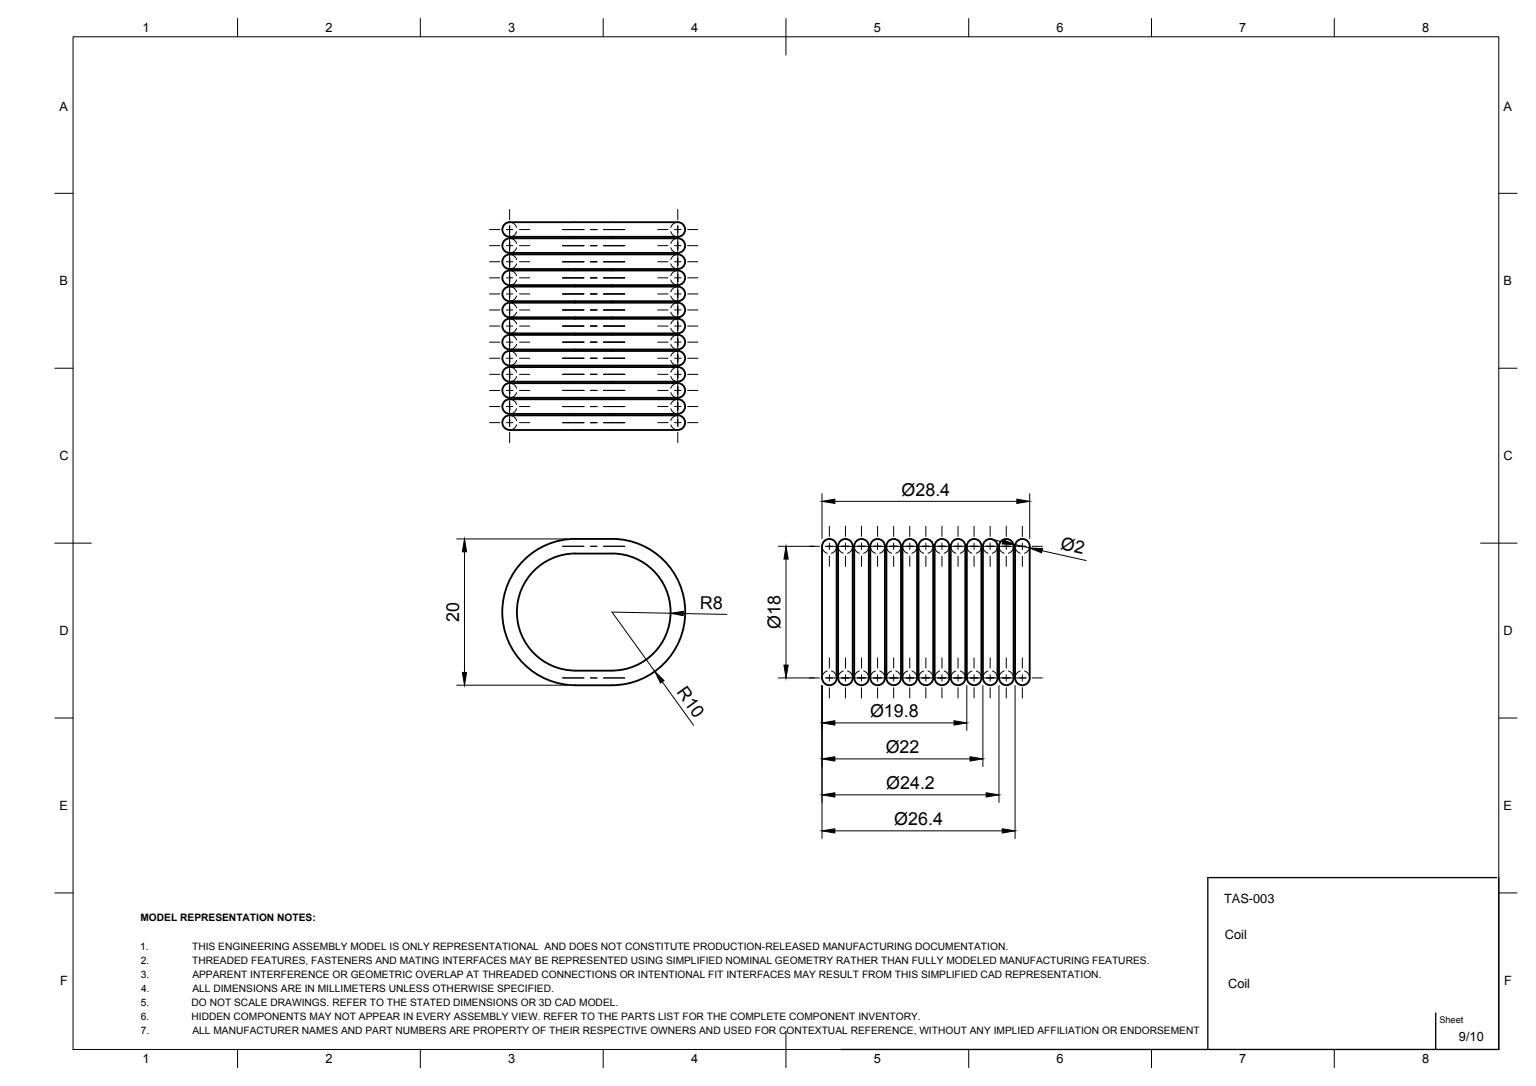
ISO-10303-21;
HEADER;
/* Generated by software containing ST-Developer
 * from STEP Tools, Inc. (www.steptools.com) 
 */

FILE_DESCRIPTION(
/* description */ ('STEP AP214'),
/* implementation_level */ '2;1');

FILE_NAME(
/* name */ 'coil.step',
/* time_stamp */ '2026-11-04T19:43:37-08:00',
/* author */ (''),
/* organization */ (''),
/* preprocessor_version */ 'ST-DEVELOPER v20.2',
/* originating_system */ 'Autodesk Translation Framework v15.17.0.0',
/* authorisation */ '');

FILE_SCHEMA (('AUTOMOTIVE_DESIGN { 1 0 10303 214 3 1 1 }'));
ENDSEC;

DATA;
#10=MECHANICAL_DESIGN_GEOMETRIC_PRESENTATION_REPRESENTATION('',(#121,#122,#123,#124,#125,#126,#127,#128,#129,#130,#131,#132,#133),#7627);
#60=TOROIDAL_SURFACE('',#2646,9.,0.999999999999999);
#61=TOROIDAL_SURFACE('',#2650,9.,0.999999999999999);
#62=TOROIDAL_SURFACE('',#2656,9.,0.999999999999999);
#63=TOROIDAL_SURFACE('',#2660,9.,0.999999999999999);
#64=TOROIDAL_SURFACE('',#2666,9.,0.999999999999999);
#65=TOROIDAL_SURFACE('',#2670,9.,0.999999999999999);
#66=TOROIDAL_SURFACE('',#2676,9.,0.999999999999999);
#67=TOROIDAL_SURFACE('',#2680,9.,0.999999999999999);
#68=TOROIDAL_SURFACE('',#2686,9.,0.999999999999999);
#69=TOROIDAL_SURFACE('',#2690,9.,0.999999999999999);
#70=TOROIDAL_SURFACE('',#2696,9.,0.999999999999999);
#71=TOROIDAL_SURFACE('',#2700,9.,0.999999999999999);
#72=TOROIDAL_SURFACE('',#2706,9.,0.999999999999999);
#73=TOROIDAL_SURFACE('',#2710,9.,0.999999999999999);
#74=TOROIDAL_SURFACE('',#2716,9.,0.999999999999999);
#75=TOROIDAL_SURFACE('',#2720,9.,0.999999999999999);
#76=TOROIDAL_SURFACE('',#2726,9.,0.999999999999999);
#77=TOROIDAL_SURFACE('',#2730,9.,0.999999999999999);
#78=TOROIDAL_SURFACE('',#2736,9.,0.999999999999999);
#79=TOROIDAL_SURFACE('',#2740,9.,0.999999999999999);
#80=TOROIDAL_SURFACE('',#2746,9.,0.999999999999999);
#81=TOROIDAL_SURFACE('',#2750,9.,0.999999999999999);
#82=TOROIDAL_SURFACE('',#2756,9.,0.999999999999999);
#83=TOROIDAL_SURFACE('',#2760,9.,0.999999999999999);
#84=TOROIDAL_SURFACE('',#2766,9.,0.999999999999999);
#85=TOROIDAL_SURFACE('',#2770,9.,0.999999999999999);
#103=SHAPE_REPRESENTATION_RELATIONSHIP('SRR','None',#7671,#112);
#112=ADVANCED_BREP_SHAPE_REPRESENTATION('',(#142,#143,#144,#145,#146,#147,
#148,#149,#150,#151,#152,#153,#154),#7624);
#121=STYLED_ITEM('',(#7723),#142);
#122=STYLED_ITEM('',(#7723),#143);
#123=STYLED_ITEM('',(#7723),#144);
#124=STYLED_ITEM('',(#7723),#145);
#125=STYLED_ITEM('',(#7723),#146);
#126=STYLED_ITEM('',(#7723),#147);
#127=STYLED_ITEM('',(#7723),#148);
#128=STYLED_ITEM('',(#7723),#149);
#129=STYLED_ITEM('',(#7723),#150);
#130=STYLED_ITEM('',(#7723),#151);
#131=STYLED_ITEM('',(#7723),#152);
#132=STYLED_ITEM('',(#7723),#153);
#133=STYLED_ITEM('',(#7723),#154);
#142=MANIFOLD_SOLID_BREP('Body1',#2419);
#143=MANIFOLD_SOLID_BREP('Body2',#2420);
#144=MANIFOLD_SOLID_BREP('Body3',#2421);
#145=MANIFOLD_SOLID_BREP('Body4',#2422);
#146=MANIFOLD_SOLID_BREP('Body5',#2423);
#147=MANIFOLD_SOLID_BREP('Body6',#2424);
#148=MANIFOLD_SOLID_BREP('Body7',#2425);
#149=MANIFOLD_SOLID_BREP('Body8',#2426);
#150=MANIFOLD_SOLID_BREP('Body9',#2427);
#151=MANIFOLD_SOLID_BREP('Body10',#2428);
#152=MANIFOLD_SOLID_BREP('Body11',#2429);
#153=MANIFOLD_SOLID_BREP('Body12',#2430);
#154=MANIFOLD_SOLID_BREP('Body13',#2431);
#276=CYLINDRICAL_SURFACE('',#2654,0.999999999999999);
#277=CYLINDRICAL_SURFACE('',#2655,0.999999999999999);
#278=CYLINDRICAL_SURFACE('',#2664,0.999999999999999);
#279=CYLINDRICAL_SURFACE('',#2665,0.999999999999999);
#280=CYLINDRICAL_SURFACE('',#2674,0.999999999999999);
#281=CYLINDRICAL_SURFACE('',#2675,0.999999999999999);
#282=CYLINDRICAL_SURFACE('',#2684,0.999999999999999);
#283=CYLINDRICAL_SURFACE('',#2685,0.999999999999999);
#284=CYLINDRICAL_SURFACE('',#2694,0.999999999999999);
#285=CYLINDRICAL_SURFACE('',#2695,0.999999999999999);
#286=CYLINDRICAL_SURFACE('',#2704,0.999999999999999);
#287=CYLINDRICAL_SURFACE('',#2705,0.999999999999999);
#288=CYLINDRICAL_SURFACE('',#2714,0.999999999999999);
#289=CYLINDRICAL_SURFACE('',#2715,0.999999999999999);
#290=CYLINDRICAL_SURFACE('',#2724,0.999999999999999);
#291=CYLINDRICAL_SURFACE('',#2725,0.999999999999999);
#292=CYLINDRICAL_SURFACE('',#2734,0.999999999999999);
#293=CYLINDRICAL_SURFACE('',#2735,0.999999999999999);
#294=CYLINDRICAL_SURFACE('',#2744,0.999999999999999);
#295=CYLINDRICAL_SURFACE('',#2745,0.999999999999999);
#296=CYLINDRICAL_SURFACE('',#2754,0.999999999999999);
#297=CYLINDRICAL_SURFACE('',#2755,0.999999999999999);
#298=CYLINDRICAL_SURFACE('',#2764,0.999999999999999);
#299=CYLINDRICAL_SURFACE('',#2765,0.999999999999999);
#300=CYLINDRICAL_SURFACE('',#2774,0.999999999999999);
#301=CYLINDRICAL_SURFACE('',#2775,0.999999999999999);
#366=FACE_OUTER_BOUND('',#542,.T.);
#367=FACE_OUTER_BOUND('',#543,.T.);
#368=FACE_OUTER_BOUND('',#544,.T.);
#369=FACE_OUTER_BOUND('',#545,.T.);
#370=FACE_OUTER_BOUND('',#546,.T.);
#371=FACE_OUTER_BOUND('',#547,.T.);
#372=FACE_OUTER_BOUND('',#548,.T.);
#373=FACE_OUTER_BOUND('',#549,.T.);
#374=FACE_OUTER_BOUND('',#550,.T.);
#375=FACE_OUTER_BOUND('',#551,.T.);
#376=FACE_OUTER_BOUND('',#552,.T.);
#377=FACE_OUTER_BOUND('',#553,.T.);
#378=FACE_OUTER_BOUND('',#554,.T.);
#379=FACE_OUTER_BOUND('',#555,.T.);
#380=FACE_OUTER_BOUND('',#556,.T.);
#381=FACE_OUTER_BOUND('',#557,.T.);
#382=FACE_OUTER_BOUND('',#558,.T.);
#383=FACE_OUTER_BOUND('',#559,.T.);
#384=FACE_OUTER_BOUND('',#560,.T.);
#385=FACE_OUTER_BOUND('',#561,.T.);
#386=FACE_OUTER_BOUND('',#562,.T.);
#387=FACE_OUTER_BOUND('',#563,.T.);
#388=FACE_OUTER_BOUND('',#564,.T.);
#389=FACE_OUTER_BOUND('',#565,.T.);
#390=FACE_OUTER_BOUND('',#566,.T.);
#391=FACE_OUTER_BOUND('',#567,.T.);
#392=FACE_OUTER_BOUND('',#568,.T.);
#393=FACE_OUTER_BOUND('',#569,.T.);
#394=FACE_OUTER_BOUND('',#570,.T.);
#395=FACE_OUTER_BOUND('',#571,.T.);
#396=FACE_OUTER_BOUND('',#572,.T.);
#397=FACE_OUTER_BOUND('',#573,.T.);
#398=FACE_OUTER_BOUND('',#574,.T.);
#399=FACE_OUTER_BOUND('',#575,.T.);
#400=FACE_OUTER_BOUND('',#576,.T.);
#401=FACE_OUTER_BOUND('',#577,.T.);
#402=FACE_OUTER_BOUND('',#578,.T.);
#403=FACE_OUTER_BOUND('',#579,.T.);
#404=FACE_OUTER_BOUND('',#580,.T.);
#405=FACE_OUTER_BOUND('',#581,.T.);
#406=FACE_OUTER_BOUND('',#582,.T.);
#407=FACE_OUTER_BOUND('',#583,.T.);
#408=FACE_OUTER_BOUND('',#584,.T.);
#409=FACE_OUTER_BOUND('',#585,.T.);
#410=FACE_OUTER_BOUND('',#586,.T.);
#411=FACE_OUTER_BOUND('',#587,.T.);
#412=FACE_OUTER_BOUND('',#588,.T.);
#413=FACE_OUTER_BOUND('',#589,.T.);
#414=FACE_OUTER_BOUND('',#590,.T.);
#415=FACE_OUTER_BOUND('',#591,.T.);
#416=FACE_OUTER_BOUND('',#592,.T.);
#417=FACE_OUTER_BOUND('',#593,.T.);
#542=EDGE_LOOP('',(#1849,#1850,#1851,#1852));
#543=EDGE_LOOP('',(#1853,#1854,#1855,#1856));
#544=EDGE_LOOP('',(#1857,#1858,#1859,#1860));
#545=EDGE_LOOP('',(#1861,#1862,#1863,#1864));
#546=EDGE_LOOP('',(#1865,#1866,#1867,#1868));
#547=EDGE_LOOP('',(#1869,#1870,#1871,#1872));
#548=EDGE_LOOP('',(#1873,#1874,#1875,#1876));
#549=EDGE_LOOP('',(#1877,#1878,#1879,#1880));
#550=EDGE_LOOP('',(#1881,#1882,#1883,#1884));
#551=EDGE_LOOP('',(#1885,#1886,#1887,#1888));
#552=EDGE_LOOP('',(#1889,#1890,#1891,#1892));
#553=EDGE_LOOP('',(#1893,#1894,#1895,#1896));
#554=EDGE_LOOP('',(#1897,#1898,#1899,#1900));
#555=EDGE_LOOP('',(#1901,#1902,#1903,#1904));
#556=EDGE_LOOP('',(#1905,#1906,#1907,#1908));
#557=EDGE_LOOP('',(#1909,#1910,#1911,#1912));
#558=EDGE_LOOP('',(#1913,#1914,#1915,#1916));
#559=EDGE_LOOP('',(#1917,#1918,#1919,#1920));
#560=EDGE_LOOP('',(#1921,#1922,#1923,#1924));
#561=EDGE_LOOP('',(#1925,#1926,#1927,#1928));
#562=EDGE_LOOP('',(#1929,#1930,#1931,#1932));
#563=EDGE_LOOP('',(#1933,#1934,#1935,#1936));
#564=EDGE_LOOP('',(#1937,#1938,#1939,#1940));
#565=EDGE_LOOP('',(#1941,#1942,#1943,#1944));
#566=EDGE_LOOP('',(#1945,#1946,#1947,#1948));
#567=EDGE_LOOP('',(#1949,#1950,#1951,#1952));
#568=EDGE_LOOP('',(#1953,#1954,#1955,#1956));
#569=EDGE_LOOP('',(#1957,#1958,#1959,#1960));
#570=EDGE_LOOP('',(#1961,#1962,#1963,#1964));
#571=EDGE_LOOP('',(#1965,#1966,#1967,#1968));
#572=EDGE_LOOP('',(#1969,#1970,#1971,#1972));
#573=EDGE_LOOP('',(#1973,#1974,#1975,#1976));
#574=EDGE_LOOP('',(#1977,#1978,#1979,#1980));
#575=EDGE_LOOP('',(#1981,#1982,#1983,#1984));
#576=EDGE_LOOP('',(#1985,#1986,#1987,#1988));
#577=EDGE_LOOP('',(#1989,#1990,#1991,#1992));
#578=EDGE_LOOP('',(#1993,#1994,#1995,#1996));
#579=EDGE_LOOP('',(#1997,#1998,#1999,#2000));
#580=EDGE_LOOP('',(#2001,#2002,#2003,#2004));
#581=EDGE_LOOP('',(#2005,#2006,#2007,#2008));
#582=EDGE_LOOP('',(#2009,#2010,#2011,#2012));
#583=EDGE_LOOP('',(#2013,#2014,#2015,#2016));
#584=EDGE_LOOP('',(#2017,#2018,#2019,#2020));
#585=EDGE_LOOP('',(#2021,#2022,#2023,#2024));
#586=EDGE_LOOP('',(#2025,#2026,#2027,#2028));
#587=EDGE_LOOP('',(#2029,#2030,#2031,#2032));
#588=EDGE_LOOP('',(#2033,#2034,#2035,#2036));
#589=EDGE_LOOP('',(#2037,#2038,#2039,#2040));
#590=EDGE_LOOP('',(#2041,#2042,#2043,#2044));
#591=EDGE_LOOP('',(#2045,#2046,#2047,#2048));
#592=EDGE_LOOP('',(#2049,#2050,#2051,#2052));
#593=EDGE_LOOP('',(#2053,#2054,#2055,#2056));
#695=CIRCLE('',#2647,0.999999999999999);
#696=CIRCLE('',#2648,8.00000000000001);
#697=CIRCLE('',#2649,0.999999999999999);
#698=CIRCLE('',#2651,0.999999999999999);
#699=CIRCLE('',#2652,8.);
#700=CIRCLE('',#2653,0.999999999999999);
#701=CIRCLE('',#2657,0.999999999999999);
#702=CIRCLE('',#2658,8.00000000000001);
#703=CIRCLE('',#2659,0.999999999999999);
#704=CIRCLE('',#2661,0.999999999999999);
#705=CIRCLE('',#2662,8.);
#706=CIRCLE('',#2663,0.999999999999999);
#707=CIRCLE('',#2667,0.999999999999999);
#708=CIRCLE('',#2668,8.00000000000001);
#709=CIRCLE('',#2669,0.999999999999999);
#710=CIRCLE('',#2671,0.999999999999999);
#711=CIRCLE('',#2672,8.);
#712=CIRCLE('',#2673,0.999999999999999);
#713=CIRCLE('',#2677,0.999999999999999);
#714=CIRCLE('',#2678,8.00000000000001);
#715=CIRCLE('',#2679,0.999999999999999);
#716=CIRCLE('',#2681,0.999999999999999);
#717=CIRCLE('',#2682,8.);
#718=CIRCLE('',#2683,0.999999999999999);
#719=CIRCLE('',#2687,0.999999999999999);
#720=CIRCLE('',#2688,8.00000000000001);
#721=CIRCLE('',#2689,0.999999999999999);
#722=CIRCLE('',#2691,0.999999999999999);
#723=CIRCLE('',#2692,8.);
#724=CIRCLE('',#2693,0.999999999999999);
#725=CIRCLE('',#2697,0.999999999999999);
#726=CIRCLE('',#2698,8.00000000000001);
#727=CIRCLE('',#2699,0.999999999999999);
#728=CIRCLE('',#2701,0.999999999999999);
#729=CIRCLE('',#2702,8.);
#730=CIRCLE('',#2703,0.999999999999999);
#731=CIRCLE('',#2707,0.999999999999999);
#732=CIRCLE('',#2708,8.00000000000001);
#733=CIRCLE('',#2709,0.999999999999999);
#734=CIRCLE('',#2711,0.999999999999999);
#735=CIRCLE('',#2712,8.);
#736=CIRCLE('',#2713,0.999999999999999);
#737=CIRCLE('',#2717,0.999999999999999);
#738=CIRCLE('',#2718,8.00000000000001);
#739=CIRCLE('',#2719,0.999999999999999);
#740=CIRCLE('',#2721,0.999999999999999);
#741=CIRCLE('',#2722,8.);
#742=CIRCLE('',#2723,0.999999999999999);
#743=CIRCLE('',#2727,0.999999999999999);
#744=CIRCLE('',#2728,8.00000000000001);
#745=CIRCLE('',#2729,0.999999999999999);
#746=CIRCLE('',#2731,0.999999999999999);
#747=CIRCLE('',#2732,8.);
#748=CIRCLE('',#2733,0.999999999999999);
#749=CIRCLE('',#2737,0.999999999999999);
#750=CIRCLE('',#2738,8.00000000000001);
#751=CIRCLE('',#2739,0.999999999999999);
#752=CIRCLE('',#2741,0.999999999999999);
#753=CIRCLE('',#2742,8.);
#754=CIRCLE('',#2743,0.999999999999999);
#755=CIRCLE('',#2747,0.999999999999999);
#756=CIRCLE('',#2748,8.00000000000001);
#757=CIRCLE('',#2749,0.999999999999999);
#758=CIRCLE('',#2751,0.999999999999999);
#759=CIRCLE('',#2752,8.);
#760=CIRCLE('',#2753,0.999999999999999);
#761=CIRCLE('',#2757,0.999999999999999);
#762=CIRCLE('',#2758,8.00000000000001);
#763=CIRCLE('',#2759,0.999999999999999);
#764=CIRCLE('',#2761,0.999999999999999);
#765=CIRCLE('',#2762,8.);
#766=CIRCLE('',#2763,0.999999999999999);
#767=CIRCLE('',#2767,0.999999999999999);
#768=CIRCLE('',#2768,8.00000000000001);
#769=CIRCLE('',#2769,0.999999999999999);
#770=CIRCLE('',#2771,0.999999999999999);
#771=CIRCLE('',#2772,8.);
#772=CIRCLE('',#2773,0.999999999999999);
#865=LINE('',#7193,#1021);
#866=LINE('',#7195,#1022);
#867=LINE('',#7209,#1023);
#868=LINE('',#7211,#1024);
#869=LINE('',#7225,#1025);
#870=LINE('',#7227,#1026);
#871=LINE('',#7241,#1027);
#872=LINE('',#7243,#1028);
#873=LINE('',#7257,#1029);
#874=LINE('',#7259,#1030);
#875=LINE('',#7273,#1031);
#876=LINE('',#7275,#1032);
#877=LINE('',#7289,#1033);
#878=LINE('',#7291,#1034);
#879=LINE('',#7305,#1035);
#880=LINE('',#7307,#1036);
#881=LINE('',#7321,#1037);
#882=LINE('',#7323,#1038);
#883=LINE('',#7337,#1039);
#884=LINE('',#7339,#1040);
#885=LINE('',#7353,#1041);
#886=LINE('',#7355,#1042);
#887=LINE('',#7369,#1043);
#888=LINE('',#7371,#1044);
#889=LINE('',#7385,#1045);
#890=LINE('',#7387,#1046);
#1021=VECTOR('',#3168,0.999999999999999);
#1022=VECTOR('',#3171,0.999999999999999);
#1023=VECTOR('',#3190,0.999999999999999);
#1024=VECTOR('',#3193,0.999999999999999);
#1025=VECTOR('',#3212,0.999999999999999);
#1026=VECTOR('',#3215,0.999999999999999);
#1027=VECTOR('',#3234,0.999999999999999);
#1028=VECTOR('',#3237,0.999999999999999);
#1029=VECTOR('',#3256,0.999999999999999);
#1030=VECTOR('',#3259,0.999999999999999);
#1031=VECTOR('',#3278,0.999999999999999);
#1032=VECTOR('',#3281,0.999999999999999);
#1033=VECTOR('',#3300,0.999999999999999);
#1034=VECTOR('',#3303,0.999999999999999);
#1035=VECTOR('',#3322,0.999999999999999);
#1036=VECTOR('',#3325,0.999999999999999);
#1037=VECTOR('',#3344,0.999999999999999);
#1038=VECTOR('',#3347,0.999999999999999);
#1039=VECTOR('',#3366,0.999999999999999);
#1040=VECTOR('',#3369,0.999999999999999);
#1041=VECTOR('',#3388,0.999999999999999);
#1042=VECTOR('',#3391,0.999999999999999);
#1043=VECTOR('',#3410,0.999999999999999);
#1044=VECTOR('',#3413,0.999999999999999);
#1045=VECTOR('',#3432,0.999999999999999);
#1046=VECTOR('',#3435,0.999999999999999);
#1191=VERTEX_POINT('',#7181);
#1192=VERTEX_POINT('',#7183);
#1193=VERTEX_POINT('',#7187);
#1194=VERTEX_POINT('',#7189);
#1195=VERTEX_POINT('',#7197);
#1196=VERTEX_POINT('',#7199);
#1197=VERTEX_POINT('',#7203);
#1198=VERTEX_POINT('',#7205);
#1199=VERTEX_POINT('',#7213);
#1200=VERTEX_POINT('',#7215);
#1201=VERTEX_POINT('',#7219);
#1202=VERTEX_POINT('',#7221);
#1203=VERTEX_POINT('',#7229);
#1204=VERTEX_POINT('',#7231);
#1205=VERTEX_POINT('',#7235);
#1206=VERTEX_POINT('',#7237);
#1207=VERTEX_POINT('',#7245);
#1208=VERTEX_POINT('',#7247);
#1209=VERTEX_POINT('',#7251);
#1210=VERTEX_POINT('',#7253);
#1211=VERTEX_POINT('',#7261);
#1212=VERTEX_POINT('',#7263);
#1213=VERTEX_POINT('',#7267);
#1214=VERTEX_POINT('',#7269);
#1215=VERTEX_POINT('',#7277);
#1216=VERTEX_POINT('',#7279);
#1217=VERTEX_POINT('',#7283);
#1218=VERTEX_POINT('',#7285);
#1219=VERTEX_POINT('',#7293);
#1220=VERTEX_POINT('',#7295);
#1221=VERTEX_POINT('',#7299);
#1222=VERTEX_POINT('',#7301);
#1223=VERTEX_POINT('',#7309);
#1224=VERTEX_POINT('',#7311);
#1225=VERTEX_POINT('',#7315);
#1226=VERTEX_POINT('',#7317);
#1227=VERTEX_POINT('',#7325);
#1228=VERTEX_POINT('',#7327);
#1229=VERTEX_POINT('',#7331);
#1230=VERTEX_POINT('',#7333);
#1231=VERTEX_POINT('',#7341);
#1232=VERTEX_POINT('',#7343);
#1233=VERTEX_POINT('',#7347);
#1234=VERTEX_POINT('',#7349);
#1235=VERTEX_POINT('',#7357);
#1236=VERTEX_POINT('',#7359);
#1237=VERTEX_POINT('',#7363);
#1238=VERTEX_POINT('',#7365);
#1239=VERTEX_POINT('',#7373);
#1240=VERTEX_POINT('',#7375);
#1241=VERTEX_POINT('',#7379);
#1242=VERTEX_POINT('',#7381);
#1419=EDGE_CURVE('',#1191,#1191,#695,.T.);
#1420=EDGE_CURVE('',#1191,#1192,#696,.T.);
#1421=EDGE_CURVE('',#1192,#1192,#697,.T.);
#1422=EDGE_CURVE('',#1193,#1193,#698,.T.);
#1423=EDGE_CURVE('',#1193,#1194,#699,.T.);
#1424=EDGE_CURVE('',#1194,#1194,#700,.T.);
#1425=EDGE_CURVE('',#1194,#1191,#865,.T.);
#1426=EDGE_CURVE('',#1192,#1193,#866,.T.);
#1427=EDGE_CURVE('',#1195,#1195,#701,.T.);
#1428=EDGE_CURVE('',#1195,#1196,#702,.T.);
#1429=EDGE_CURVE('',#1196,#1196,#703,.T.);
#1430=EDGE_CURVE('',#1197,#1197,#704,.T.);
#1431=EDGE_CURVE('',#1197,#1198,#705,.T.);
#1432=EDGE_CURVE('',#1198,#1198,#706,.T.);
#1433=EDGE_CURVE('',#1198,#1195,#867,.T.);
#1434=EDGE_CURVE('',#1196,#1197,#868,.T.);
#1435=EDGE_CURVE('',#1199,#1199,#707,.T.);
#1436=EDGE_CURVE('',#1199,#1200,#708,.T.);
#1437=EDGE_CURVE('',#1200,#1200,#709,.T.);
#1438=EDGE_CURVE('',#1201,#1201,#710,.T.);
#1439=EDGE_CURVE('',#1201,#1202,#711,.T.);
#1440=EDGE_CURVE('',#1202,#1202,#712,.T.);
#1441=EDGE_CURVE('',#1202,#1199,#869,.T.);
#1442=EDGE_CURVE('',#1200,#1201,#870,.T.);
#1443=EDGE_CURVE('',#1203,#1203,#713,.T.);
#1444=EDGE_CURVE('',#1203,#1204,#714,.T.);
#1445=EDGE_CURVE('',#1204,#1204,#715,.T.);
#1446=EDGE_CURVE('',#1205,#1205,#716,.T.);
#1447=EDGE_CURVE('',#1205,#1206,#717,.T.);
#1448=EDGE_CURVE('',#1206,#1206,#718,.T.);
#1449=EDGE_CURVE('',#1206,#1203,#871,.T.);
#1450=EDGE_CURVE('',#1204,#1205,#872,.T.);
#1451=EDGE_CURVE('',#1207,#1207,#719,.T.);
#1452=EDGE_CURVE('',#1207,#1208,#720,.T.);
#1453=EDGE_CURVE('',#1208,#1208,#721,.T.);
#1454=EDGE_CURVE('',#1209,#1209,#722,.T.);
#1455=EDGE_CURVE('',#1209,#1210,#723,.T.);
#1456=EDGE_CURVE('',#1210,#1210,#724,.T.);
#1457=EDGE_CURVE('',#1210,#1207,#873,.T.);
#1458=EDGE_CURVE('',#1208,#1209,#874,.T.);
#1459=EDGE_CURVE('',#1211,#1211,#725,.T.);
#1460=EDGE_CURVE('',#1211,#1212,#726,.T.);
#1461=EDGE_CURVE('',#1212,#1212,#727,.T.);
#1462=EDGE_CURVE('',#1213,#1213,#728,.T.);
#1463=EDGE_CURVE('',#1213,#1214,#729,.T.);
#1464=EDGE_CURVE('',#1214,#1214,#730,.T.);
#1465=EDGE_CURVE('',#1214,#1211,#875,.T.);
#1466=EDGE_CURVE('',#1212,#1213,#876,.T.);
#1467=EDGE_CURVE('',#1215,#1215,#731,.T.);
#1468=EDGE_CURVE('',#1215,#1216,#732,.T.);
#1469=EDGE_CURVE('',#1216,#1216,#733,.T.);
#1470=EDGE_CURVE('',#1217,#1217,#734,.T.);
#1471=EDGE_CURVE('',#1217,#1218,#735,.T.);
#1472=EDGE_CURVE('',#1218,#1218,#736,.T.);
#1473=EDGE_CURVE('',#1218,#1215,#877,.T.);
#1474=EDGE_CURVE('',#1216,#1217,#878,.T.);
#1475=EDGE_CURVE('',#1219,#1219,#737,.T.);
#1476=EDGE_CURVE('',#1219,#1220,#738,.T.);
#1477=EDGE_CURVE('',#1220,#1220,#739,.T.);
#1478=EDGE_CURVE('',#1221,#1221,#740,.T.);
#1479=EDGE_CURVE('',#1221,#1222,#741,.T.);
#1480=EDGE_CURVE('',#1222,#1222,#742,.T.);
#1481=EDGE_CURVE('',#1222,#1219,#879,.T.);
#1482=EDGE_CURVE('',#1220,#1221,#880,.T.);
#1483=EDGE_CURVE('',#1223,#1223,#743,.T.);
#1484=EDGE_CURVE('',#1223,#1224,#744,.T.);
#1485=EDGE_CURVE('',#1224,#1224,#745,.T.);
#1486=EDGE_CURVE('',#1225,#1225,#746,.T.);
#1487=EDGE_CURVE('',#1225,#1226,#747,.T.);
#1488=EDGE_CURVE('',#1226,#1226,#748,.T.);
#1489=EDGE_CURVE('',#1226,#1223,#881,.T.);
#1490=EDGE_CURVE('',#1224,#1225,#882,.T.);
#1491=EDGE_CURVE('',#1227,#1227,#749,.T.);
#1492=EDGE_CURVE('',#1227,#1228,#750,.T.);
#1493=EDGE_CURVE('',#1228,#1228,#751,.T.);
#1494=EDGE_CURVE('',#1229,#1229,#752,.T.);
#1495=EDGE_CURVE('',#1229,#1230,#753,.T.);
#1496=EDGE_CURVE('',#1230,#1230,#754,.T.);
#1497=EDGE_CURVE('',#1230,#1227,#883,.T.);
#1498=EDGE_CURVE('',#1228,#1229,#884,.T.);
#1499=EDGE_CURVE('',#1231,#1231,#755,.T.);
#1500=EDGE_CURVE('',#1231,#1232,#756,.T.);
#1501=EDGE_CURVE('',#1232,#1232,#757,.T.);
#1502=EDGE_CURVE('',#1233,#1233,#758,.T.);
#1503=EDGE_CURVE('',#1233,#1234,#759,.T.);
#1504=EDGE_CURVE('',#1234,#1234,#760,.T.);
#1505=EDGE_CURVE('',#1234,#1231,#885,.T.);
#1506=EDGE_CURVE('',#1232,#1233,#886,.T.);
#1507=EDGE_CURVE('',#1235,#1235,#761,.T.);
#1508=EDGE_CURVE('',#1235,#1236,#762,.T.);
#1509=EDGE_CURVE('',#1236,#1236,#763,.T.);
#1510=EDGE_CURVE('',#1237,#1237,#764,.T.);
#1511=EDGE_CURVE('',#1237,#1238,#765,.T.);
#1512=EDGE_CURVE('',#1238,#1238,#766,.T.);
#1513=EDGE_CURVE('',#1238,#1235,#887,.T.);
#1514=EDGE_CURVE('',#1236,#1237,#888,.T.);
#1515=EDGE_CURVE('',#1239,#1239,#767,.T.);
#1516=EDGE_CURVE('',#1239,#1240,#768,.T.);
#1517=EDGE_CURVE('',#1240,#1240,#769,.T.);
#1518=EDGE_CURVE('',#1241,#1241,#770,.T.);
#1519=EDGE_CURVE('',#1241,#1242,#771,.T.);
#1520=EDGE_CURVE('',#1242,#1242,#772,.T.);
#1521=EDGE_CURVE('',#1242,#1239,#889,.T.);
#1522=EDGE_CURVE('',#1240,#1241,#890,.T.);
#1849=ORIENTED_EDGE('',*,*,#1419,.T.);
#1850=ORIENTED_EDGE('',*,*,#1420,.T.);
#1851=ORIENTED_EDGE('',*,*,#1421,.F.);
#1852=ORIENTED_EDGE('',*,*,#1420,.F.);
#1853=ORIENTED_EDGE('',*,*,#1422,.T.);
#1854=ORIENTED_EDGE('',*,*,#1423,.T.);
#1855=ORIENTED_EDGE('',*,*,#1424,.F.);
#1856=ORIENTED_EDGE('',*,*,#1423,.F.);
#1857=ORIENTED_EDGE('',*,*,#1424,.T.);
#1858=ORIENTED_EDGE('',*,*,#1425,.T.);
#1859=ORIENTED_EDGE('',*,*,#1419,.F.);
#1860=ORIENTED_EDGE('',*,*,#1425,.F.);
#1861=ORIENTED_EDGE('',*,*,#1421,.T.);
#1862=ORIENTED_EDGE('',*,*,#1426,.T.);
#1863=ORIENTED_EDGE('',*,*,#1422,.F.);
#1864=ORIENTED_EDGE('',*,*,#1426,.F.);
#1865=ORIENTED_EDGE('',*,*,#1427,.T.);
#1866=ORIENTED_EDGE('',*,*,#1428,.T.);
#1867=ORIENTED_EDGE('',*,*,#1429,.F.);
#1868=ORIENTED_EDGE('',*,*,#1428,.F.);
#1869=ORIENTED_EDGE('',*,*,#1430,.T.);
#1870=ORIENTED_EDGE('',*,*,#1431,.T.);
#1871=ORIENTED_EDGE('',*,*,#1432,.F.);
#1872=ORIENTED_EDGE('',*,*,#1431,.F.);
#1873=ORIENTED_EDGE('',*,*,#1432,.T.);
#1874=ORIENTED_EDGE('',*,*,#1433,.T.);
#1875=ORIENTED_EDGE('',*,*,#1427,.F.);
#1876=ORIENTED_EDGE('',*,*,#1433,.F.);
#1877=ORIENTED_EDGE('',*,*,#1429,.T.);
#1878=ORIENTED_EDGE('',*,*,#1434,.T.);
#1879=ORIENTED_EDGE('',*,*,#1430,.F.);
#1880=ORIENTED_EDGE('',*,*,#1434,.F.);
#1881=ORIENTED_EDGE('',*,*,#1435,.T.);
#1882=ORIENTED_EDGE('',*,*,#1436,.T.);
#1883=ORIENTED_EDGE('',*,*,#1437,.F.);
#1884=ORIENTED_EDGE('',*,*,#1436,.F.);
#1885=ORIENTED_EDGE('',*,*,#1438,.T.);
#1886=ORIENTED_EDGE('',*,*,#1439,.T.);
#1887=ORIENTED_EDGE('',*,*,#1440,.F.);
#1888=ORIENTED_EDGE('',*,*,#1439,.F.);
#1889=ORIENTED_EDGE('',*,*,#1440,.T.);
#1890=ORIENTED_EDGE('',*,*,#1441,.T.);
#1891=ORIENTED_EDGE('',*,*,#1435,.F.);
#1892=ORIENTED_EDGE('',*,*,#1441,.F.);
#1893=ORIENTED_EDGE('',*,*,#1437,.T.);
#1894=ORIENTED_EDGE('',*,*,#1442,.T.);
#1895=ORIENTED_EDGE('',*,*,#1438,.F.);
#1896=ORIENTED_EDGE('',*,*,#1442,.F.);
#1897=ORIENTED_EDGE('',*,*,#1443,.T.);
#1898=ORIENTED_EDGE('',*,*,#1444,.T.);
#1899=ORIENTED_EDGE('',*,*,#1445,.F.);
#1900=ORIENTED_EDGE('',*,*,#1444,.F.);
#1901=ORIENTED_EDGE('',*,*,#1446,.T.);
#1902=ORIENTED_EDGE('',*,*,#1447,.T.);
#1903=ORIENTED_EDGE('',*,*,#1448,.F.);
#1904=ORIENTED_EDGE('',*,*,#1447,.F.);
#1905=ORIENTED_EDGE('',*,*,#1448,.T.);
#1906=ORIENTED_EDGE('',*,*,#1449,.T.);
#1907=ORIENTED_EDGE('',*,*,#1443,.F.);
#1908=ORIENTED_EDGE('',*,*,#1449,.F.);
#1909=ORIENTED_EDGE('',*,*,#1445,.T.);
#1910=ORIENTED_EDGE('',*,*,#1450,.T.);
#1911=ORIENTED_EDGE('',*,*,#1446,.F.);
#1912=ORIENTED_EDGE('',*,*,#1450,.F.);
#1913=ORIENTED_EDGE('',*,*,#1451,.T.);
#1914=ORIENTED_EDGE('',*,*,#1452,.T.);
#1915=ORIENTED_EDGE('',*,*,#1453,.F.);
#1916=ORIENTED_EDGE('',*,*,#1452,.F.);
#1917=ORIENTED_EDGE('',*,*,#1454,.T.);
#1918=ORIENTED_EDGE('',*,*,#1455,.T.);
#1919=ORIENTED_EDGE('',*,*,#1456,.F.);
#1920=ORIENTED_EDGE('',*,*,#1455,.F.);
#1921=ORIENTED_EDGE('',*,*,#1456,.T.);
#1922=ORIENTED_EDGE('',*,*,#1457,.T.);
#1923=ORIENTED_EDGE('',*,*,#1451,.F.);
#1924=ORIENTED_EDGE('',*,*,#1457,.F.);
#1925=ORIENTED_EDGE('',*,*,#1453,.T.);
#1926=ORIENTED_EDGE('',*,*,#1458,.T.);
#1927=ORIENTED_EDGE('',*,*,#1454,.F.);
#1928=ORIENTED_EDGE('',*,*,#1458,.F.);
#1929=ORIENTED_EDGE('',*,*,#1459,.T.);
#1930=ORIENTED_EDGE('',*,*,#1460,.T.);
#1931=ORIENTED_EDGE('',*,*,#1461,.F.);
#1932=ORIENTED_EDGE('',*,*,#1460,.F.);
#1933=ORIENTED_EDGE('',*,*,#1462,.T.);
#1934=ORIENTED_EDGE('',*,*,#1463,.T.);
#1935=ORIENTED_EDGE('',*,*,#1464,.F.);
#1936=ORIENTED_EDGE('',*,*,#1463,.F.);
#1937=ORIENTED_EDGE('',*,*,#1464,.T.);
#1938=ORIENTED_EDGE('',*,*,#1465,.T.);
#1939=ORIENTED_EDGE('',*,*,#1459,.F.);
#1940=ORIENTED_EDGE('',*,*,#1465,.F.);
#1941=ORIENTED_EDGE('',*,*,#1461,.T.);
#1942=ORIENTED_EDGE('',*,*,#1466,.T.);
#1943=ORIENTED_EDGE('',*,*,#1462,.F.);
#1944=ORIENTED_EDGE('',*,*,#1466,.F.);
#1945=ORIENTED_EDGE('',*,*,#1467,.T.);
#1946=ORIENTED_EDGE('',*,*,#1468,.T.);
#1947=ORIENTED_EDGE('',*,*,#1469,.F.);
#1948=ORIENTED_EDGE('',*,*,#1468,.F.);
#1949=ORIENTED_EDGE('',*,*,#1470,.T.);
#1950=ORIENTED_EDGE('',*,*,#1471,.T.);
#1951=ORIENTED_EDGE('',*,*,#1472,.F.);
#1952=ORIENTED_EDGE('',*,*,#1471,.F.);
#1953=ORIENTED_EDGE('',*,*,#1472,.T.);
#1954=ORIENTED_EDGE('',*,*,#1473,.T.);
#1955=ORIENTED_EDGE('',*,*,#1467,.F.);
#1956=ORIENTED_EDGE('',*,*,#1473,.F.);
#1957=ORIENTED_EDGE('',*,*,#1469,.T.);
#1958=ORIENTED_EDGE('',*,*,#1474,.T.);
#1959=ORIENTED_EDGE('',*,*,#1470,.F.);
#1960=ORIENTED_EDGE('',*,*,#1474,.F.);
#1961=ORIENTED_EDGE('',*,*,#1475,.T.);
#1962=ORIENTED_EDGE('',*,*,#1476,.T.);
#1963=ORIENTED_EDGE('',*,*,#1477,.F.);
#1964=ORIENTED_EDGE('',*,*,#1476,.F.);
#1965=ORIENTED_EDGE('',*,*,#1478,.T.);
#1966=ORIENTED_EDGE('',*,*,#1479,.T.);
#1967=ORIENTED_EDGE('',*,*,#1480,.F.);
#1968=ORIENTED_EDGE('',*,*,#1479,.F.);
#1969=ORIENTED_EDGE('',*,*,#1480,.T.);
#1970=ORIENTED_EDGE('',*,*,#1481,.T.);
#1971=ORIENTED_EDGE('',*,*,#1475,.F.);
#1972=ORIENTED_EDGE('',*,*,#1481,.F.);
#1973=ORIENTED_EDGE('',*,*,#1477,.T.);
#1974=ORIENTED_EDGE('',*,*,#1482,.T.);
#1975=ORIENTED_EDGE('',*,*,#1478,.F.);
#1976=ORIENTED_EDGE('',*,*,#1482,.F.);
#1977=ORIENTED_EDGE('',*,*,#1483,.T.);
#1978=ORIENTED_EDGE('',*,*,#1484,.T.);
#1979=ORIENTED_EDGE('',*,*,#1485,.F.);
#1980=ORIENTED_EDGE('',*,*,#1484,.F.);
#1981=ORIENTED_EDGE('',*,*,#1486,.T.);
#1982=ORIENTED_EDGE('',*,*,#1487,.T.);
#1983=ORIENTED_EDGE('',*,*,#1488,.F.);
#1984=ORIENTED_EDGE('',*,*,#1487,.F.);
#1985=ORIENTED_EDGE('',*,*,#1488,.T.);
#1986=ORIENTED_EDGE('',*,*,#1489,.T.);
#1987=ORIENTED_EDGE('',*,*,#1483,.F.);
#1988=ORIENTED_EDGE('',*,*,#1489,.F.);
#1989=ORIENTED_EDGE('',*,*,#1485,.T.);
#1990=ORIENTED_EDGE('',*,*,#1490,.T.);
#1991=ORIENTED_EDGE('',*,*,#1486,.F.);
#1992=ORIENTED_EDGE('',*,*,#1490,.F.);
#1993=ORIENTED_EDGE('',*,*,#1491,.T.);
#1994=ORIENTED_EDGE('',*,*,#1492,.T.);
#1995=ORIENTED_EDGE('',*,*,#1493,.F.);
#1996=ORIENTED_EDGE('',*,*,#1492,.F.);
#1997=ORIENTED_EDGE('',*,*,#1494,.T.);
#1998=ORIENTED_EDGE('',*,*,#1495,.T.);
#1999=ORIENTED_EDGE('',*,*,#1496,.F.);
#2000=ORIENTED_EDGE('',*,*,#1495,.F.);
#2001=ORIENTED_EDGE('',*,*,#1496,.T.);
#2002=ORIENTED_EDGE('',*,*,#1497,.T.);
#2003=ORIENTED_EDGE('',*,*,#1491,.F.);
#2004=ORIENTED_EDGE('',*,*,#1497,.F.);
#2005=ORIENTED_EDGE('',*,*,#1493,.T.);
#2006=ORIENTED_EDGE('',*,*,#1498,.T.);
#2007=ORIENTED_EDGE('',*,*,#1494,.F.);
#2008=ORIENTED_EDGE('',*,*,#1498,.F.);
#2009=ORIENTED_EDGE('',*,*,#1499,.T.);
#2010=ORIENTED_EDGE('',*,*,#1500,.T.);
#2011=ORIENTED_EDGE('',*,*,#1501,.F.);
#2012=ORIENTED_EDGE('',*,*,#1500,.F.);
#2013=ORIENTED_EDGE('',*,*,#1502,.T.);
#2014=ORIENTED_EDGE('',*,*,#1503,.T.);
#2015=ORIENTED_EDGE('',*,*,#1504,.F.);
#2016=ORIENTED_EDGE('',*,*,#1503,.F.);
#2017=ORIENTED_EDGE('',*,*,#1504,.T.);
#2018=ORIENTED_EDGE('',*,*,#1505,.T.);
#2019=ORIENTED_EDGE('',*,*,#1499,.F.);
#2020=ORIENTED_EDGE('',*,*,#1505,.F.);
#2021=ORIENTED_EDGE('',*,*,#1501,.T.);
#2022=ORIENTED_EDGE('',*,*,#1506,.T.);
#2023=ORIENTED_EDGE('',*,*,#1502,.F.);
#2024=ORIENTED_EDGE('',*,*,#1506,.F.);
#2025=ORIENTED_EDGE('',*,*,#1507,.T.);
#2026=ORIENTED_EDGE('',*,*,#1508,.T.);
#2027=ORIENTED_EDGE('',*,*,#1509,.F.);
#2028=ORIENTED_EDGE('',*,*,#1508,.F.);
#2029=ORIENTED_EDGE('',*,*,#1510,.T.);
#2030=ORIENTED_EDGE('',*,*,#1511,.T.);
#2031=ORIENTED_EDGE('',*,*,#1512,.F.);
#2032=ORIENTED_EDGE('',*,*,#1511,.F.);
#2033=ORIENTED_EDGE('',*,*,#1512,.T.);
#2034=ORIENTED_EDGE('',*,*,#1513,.T.);
#2035=ORIENTED_EDGE('',*,*,#1507,.F.);
#2036=ORIENTED_EDGE('',*,*,#1513,.F.);
#2037=ORIENTED_EDGE('',*,*,#1509,.T.);
#2038=ORIENTED_EDGE('',*,*,#1514,.T.);
#2039=ORIENTED_EDGE('',*,*,#1510,.F.);
#2040=ORIENTED_EDGE('',*,*,#1514,.F.);
#2041=ORIENTED_EDGE('',*,*,#1515,.T.);
#2042=ORIENTED_EDGE('',*,*,#1516,.T.);
#2043=ORIENTED_EDGE('',*,*,#1517,.F.);
#2044=ORIENTED_EDGE('',*,*,#1516,.F.);
#2045=ORIENTED_EDGE('',*,*,#1518,.T.);
#2046=ORIENTED_EDGE('',*,*,#1519,.T.);
#2047=ORIENTED_EDGE('',*,*,#1520,.F.);
#2048=ORIENTED_EDGE('',*,*,#1519,.F.);
#2049=ORIENTED_EDGE('',*,*,#1520,.T.);
#2050=ORIENTED_EDGE('',*,*,#1521,.T.);
#2051=ORIENTED_EDGE('',*,*,#1515,.F.);
#2052=ORIENTED_EDGE('',*,*,#1521,.F.);
#2053=ORIENTED_EDGE('',*,*,#1517,.T.);
#2054=ORIENTED_EDGE('',*,*,#1522,.T.);
#2055=ORIENTED_EDGE('',*,*,#1518,.F.);
#2056=ORIENTED_EDGE('',*,*,#1522,.F.);
#2317=ADVANCED_FACE('',(#366),#60,.T.);
#2318=ADVANCED_FACE('',(#367),#61,.T.);
#2319=ADVANCED_FACE('',(#368),#276,.T.);
#2320=ADVANCED_FACE('',(#369),#277,.T.);
#2321=ADVANCED_FACE('',(#370),#62,.T.);
#2322=ADVANCED_FACE('',(#371),#63,.T.);
#2323=ADVANCED_FACE('',(#372),#278,.T.);
#2324=ADVANCED_FACE('',(#373),#279,.T.);
#2325=ADVANCED_FACE('',(#374),#64,.T.);
#2326=ADVANCED_FACE('',(#375),#65,.T.);
#2327=ADVANCED_FACE('',(#376),#280,.T.);
#2328=ADVANCED_FACE('',(#377),#281,.T.);
#2329=ADVANCED_FACE('',(#378),#66,.T.);
#2330=ADVANCED_FACE('',(#379),#67,.T.);
#2331=ADVANCED_FACE('',(#380),#282,.T.);
#2332=ADVANCED_FACE('',(#381),#283,.T.);
#2333=ADVANCED_FACE('',(#382),#68,.T.);
#2334=ADVANCED_FACE('',(#383),#69,.T.);
#2335=ADVANCED_FACE('',(#384),#284,.T.);
#2336=ADVANCED_FACE('',(#385),#285,.T.);
#2337=ADVANCED_FACE('',(#386),#70,.T.);
#2338=ADVANCED_FACE('',(#387),#71,.T.);
#2339=ADVANCED_FACE('',(#388),#286,.T.);
#2340=ADVANCED_FACE('',(#389),#287,.T.);
#2341=ADVANCED_FACE('',(#390),#72,.T.);
#2342=ADVANCED_FACE('',(#391),#73,.T.);
#2343=ADVANCED_FACE('',(#392),#288,.T.);
#2344=ADVANCED_FACE('',(#393),#289,.T.);
#2345=ADVANCED_FACE('',(#394),#74,.T.);
#2346=ADVANCED_FACE('',(#395),#75,.T.);
#2347=ADVANCED_FACE('',(#396),#290,.T.);
#2348=ADVANCED_FACE('',(#397),#291,.T.);
#2349=ADVANCED_FACE('',(#398),#76,.T.);
#2350=ADVANCED_FACE('',(#399),#77,.T.);
#2351=ADVANCED_FACE('',(#400),#292,.T.);
#2352=ADVANCED_FACE('',(#401),#293,.T.);
#2353=ADVANCED_FACE('',(#402),#78,.T.);
#2354=ADVANCED_FACE('',(#403),#79,.T.);
#2355=ADVANCED_FACE('',(#404),#294,.T.);
#2356=ADVANCED_FACE('',(#405),#295,.T.);
#2357=ADVANCED_FACE('',(#406),#80,.T.);
#2358=ADVANCED_FACE('',(#407),#81,.T.);
#2359=ADVANCED_FACE('',(#408),#296,.T.);
#2360=ADVANCED_FACE('',(#409),#297,.T.);
#2361=ADVANCED_FACE('',(#410),#82,.T.);
#2362=ADVANCED_FACE('',(#411),#83,.T.);
#2363=ADVANCED_FACE('',(#412),#298,.T.);
#2364=ADVANCED_FACE('',(#413),#299,.T.);
#2365=ADVANCED_FACE('',(#414),#84,.T.);
#2366=ADVANCED_FACE('',(#415),#85,.T.);
#2367=ADVANCED_FACE('',(#416),#300,.T.);
#2368=ADVANCED_FACE('',(#417),#301,.T.);
#2419=CLOSED_SHELL('',(#2317,#2318,#2319,#2320));
#2420=CLOSED_SHELL('',(#2321,#2322,#2323,#2324));
#2421=CLOSED_SHELL('',(#2325,#2326,#2327,#2328));
#2422=CLOSED_SHELL('',(#2329,#2330,#2331,#2332));
#2423=CLOSED_SHELL('',(#2333,#2334,#2335,#2336));
#2424=CLOSED_SHELL('',(#2337,#2338,#2339,#2340));
#2425=CLOSED_SHELL('',(#2341,#2342,#2343,#2344));
#2426=CLOSED_SHELL('',(#2345,#2346,#2347,#2348));
#2427=CLOSED_SHELL('',(#2349,#2350,#2351,#2352));
#2428=CLOSED_SHELL('',(#2353,#2354,#2355,#2356));
#2429=CLOSED_SHELL('',(#2357,#2358,#2359,#2360));
#2430=CLOSED_SHELL('',(#2361,#2362,#2363,#2364));
#2431=CLOSED_SHELL('',(#2365,#2366,#2367,#2368));
#2645=AXIS2_PLACEMENT_3D('',#7179,#3148,#3149);
#2646=AXIS2_PLACEMENT_3D('',#7180,#3150,#3151);
#2647=AXIS2_PLACEMENT_3D('',#7182,#3152,#3153);
#2648=AXIS2_PLACEMENT_3D('',#7184,#3154,#3155);
#2649=AXIS2_PLACEMENT_3D('',#7185,#3156,#3157);
#2650=AXIS2_PLACEMENT_3D('',#7186,#3158,#3159);
#2651=AXIS2_PLACEMENT_3D('',#7188,#3160,#3161);
#2652=AXIS2_PLACEMENT_3D('',#7190,#3162,#3163);
#2653=AXIS2_PLACEMENT_3D('',#7191,#3164,#3165);
#2654=AXIS2_PLACEMENT_3D('',#7192,#3166,#3167);
#2655=AXIS2_PLACEMENT_3D('',#7194,#3169,#3170);
#2656=AXIS2_PLACEMENT_3D('',#7196,#3172,#3173);
#2657=AXIS2_PLACEMENT_3D('',#7198,#3174,#3175);
#2658=AXIS2_PLACEMENT_3D('',#7200,#3176,#3177);
#2659=AXIS2_PLACEMENT_3D('',#7201,#3178,#3179);
#2660=AXIS2_PLACEMENT_3D('',#7202,#3180,#3181);
#2661=AXIS2_PLACEMENT_3D('',#7204,#3182,#3183);
#2662=AXIS2_PLACEMENT_3D('',#7206,#3184,#3185);
#2663=AXIS2_PLACEMENT_3D('',#7207,#3186,#3187);
#2664=AXIS2_PLACEMENT_3D('',#7208,#3188,#3189);
#2665=AXIS2_PLACEMENT_3D('',#7210,#3191,#3192);
#2666=AXIS2_PLACEMENT_3D('',#7212,#3194,#3195);
#2667=AXIS2_PLACEMENT_3D('',#7214,#3196,#3197);
#2668=AXIS2_PLACEMENT_3D('',#7216,#3198,#3199);
#2669=AXIS2_PLACEMENT_3D('',#7217,#3200,#3201);
#2670=AXIS2_PLACEMENT_3D('',#7218,#3202,#3203);
#2671=AXIS2_PLACEMENT_3D('',#7220,#3204,#3205);
#2672=AXIS2_PLACEMENT_3D('',#7222,#3206,#3207);
#2673=AXIS2_PLACEMENT_3D('',#7223,#3208,#3209);
#2674=AXIS2_PLACEMENT_3D('',#7224,#3210,#3211);
#2675=AXIS2_PLACEMENT_3D('',#7226,#3213,#3214);
#2676=AXIS2_PLACEMENT_3D('',#7228,#3216,#3217);
#2677=AXIS2_PLACEMENT_3D('',#7230,#3218,#3219);
#2678=AXIS2_PLACEMENT_3D('',#7232,#3220,#3221);
#2679=AXIS2_PLACEMENT_3D('',#7233,#3222,#3223);
#2680=AXIS2_PLACEMENT_3D('',#7234,#3224,#3225);
#2681=AXIS2_PLACEMENT_3D('',#7236,#3226,#3227);
#2682=AXIS2_PLACEMENT_3D('',#7238,#3228,#3229);
#2683=AXIS2_PLACEMENT_3D('',#7239,#3230,#3231);
#2684=AXIS2_PLACEMENT_3D('',#7240,#3232,#3233);
#2685=AXIS2_PLACEMENT_3D('',#7242,#3235,#3236);
#2686=AXIS2_PLACEMENT_3D('',#7244,#3238,#3239);
#2687=AXIS2_PLACEMENT_3D('',#7246,#3240,#3241);
#2688=AXIS2_PLACEMENT_3D('',#7248,#3242,#3243);
#2689=AXIS2_PLACEMENT_3D('',#7249,#3244,#3245);
#2690=AXIS2_PLACEMENT_3D('',#7250,#3246,#3247);
#2691=AXIS2_PLACEMENT_3D('',#7252,#3248,#3249);
#2692=AXIS2_PLACEMENT_3D('',#7254,#3250,#3251);
#2693=AXIS2_PLACEMENT_3D('',#7255,#3252,#3253);
#2694=AXIS2_PLACEMENT_3D('',#7256,#3254,#3255);
#2695=AXIS2_PLACEMENT_3D('',#7258,#3257,#3258);
#2696=AXIS2_PLACEMENT_3D('',#7260,#3260,#3261);
#2697=AXIS2_PLACEMENT_3D('',#7262,#3262,#3263);
#2698=AXIS2_PLACEMENT_3D('',#7264,#3264,#3265);
#2699=AXIS2_PLACEMENT_3D('',#7265,#3266,#3267);
#2700=AXIS2_PLACEMENT_3D('',#7266,#3268,#3269);
#2701=AXIS2_PLACEMENT_3D('',#7268,#3270,#3271);
#2702=AXIS2_PLACEMENT_3D('',#7270,#3272,#3273);
#2703=AXIS2_PLACEMENT_3D('',#7271,#3274,#3275);
#2704=AXIS2_PLACEMENT_3D('',#7272,#3276,#3277);
#2705=AXIS2_PLACEMENT_3D('',#7274,#3279,#3280);
#2706=AXIS2_PLACEMENT_3D('',#7276,#3282,#3283);
#2707=AXIS2_PLACEMENT_3D('',#7278,#3284,#3285);
#2708=AXIS2_PLACEMENT_3D('',#7280,#3286,#3287);
#2709=AXIS2_PLACEMENT_3D('',#7281,#3288,#3289);
#2710=AXIS2_PLACEMENT_3D('',#7282,#3290,#3291);
#2711=AXIS2_PLACEMENT_3D('',#7284,#3292,#3293);
#2712=AXIS2_PLACEMENT_3D('',#7286,#3294,#3295);
#2713=AXIS2_PLACEMENT_3D('',#7287,#3296,#3297);
#2714=AXIS2_PLACEMENT_3D('',#7288,#3298,#3299);
#2715=AXIS2_PLACEMENT_3D('',#7290,#3301,#3302);
#2716=AXIS2_PLACEMENT_3D('',#7292,#3304,#3305);
#2717=AXIS2_PLACEMENT_3D('',#7294,#3306,#3307);
#2718=AXIS2_PLACEMENT_3D('',#7296,#3308,#3309);
#2719=AXIS2_PLACEMENT_3D('',#7297,#3310,#3311);
#2720=AXIS2_PLACEMENT_3D('',#7298,#3312,#3313);
#2721=AXIS2_PLACEMENT_3D('',#7300,#3314,#3315);
#2722=AXIS2_PLACEMENT_3D('',#7302,#3316,#3317);
#2723=AXIS2_PLACEMENT_3D('',#7303,#3318,#3319);
#2724=AXIS2_PLACEMENT_3D('',#7304,#3320,#3321);
#2725=AXIS2_PLACEMENT_3D('',#7306,#3323,#3324);
#2726=AXIS2_PLACEMENT_3D('',#7308,#3326,#3327);
#2727=AXIS2_PLACEMENT_3D('',#7310,#3328,#3329);
#2728=AXIS2_PLACEMENT_3D('',#7312,#3330,#3331);
#2729=AXIS2_PLACEMENT_3D('',#7313,#3332,#3333);
#2730=AXIS2_PLACEMENT_3D('',#7314,#3334,#3335);
#2731=AXIS2_PLACEMENT_3D('',#7316,#3336,#3337);
#2732=AXIS2_PLACEMENT_3D('',#7318,#3338,#3339);
#2733=AXIS2_PLACEMENT_3D('',#7319,#3340,#3341);
#2734=AXIS2_PLACEMENT_3D('',#7320,#3342,#3343);
#2735=AXIS2_PLACEMENT_3D('',#7322,#3345,#3346);
#2736=AXIS2_PLACEMENT_3D('',#7324,#3348,#3349);
#2737=AXIS2_PLACEMENT_3D('',#7326,#3350,#3351);
#2738=AXIS2_PLACEMENT_3D('',#7328,#3352,#3353);
#2739=AXIS2_PLACEMENT_3D('',#7329,#3354,#3355);
#2740=AXIS2_PLACEMENT_3D('',#7330,#3356,#3357);
#2741=AXIS2_PLACEMENT_3D('',#7332,#3358,#3359);
#2742=AXIS2_PLACEMENT_3D('',#7334,#3360,#3361);
#2743=AXIS2_PLACEMENT_3D('',#7335,#3362,#3363);
#2744=AXIS2_PLACEMENT_3D('',#7336,#3364,#3365);
#2745=AXIS2_PLACEMENT_3D('',#7338,#3367,#3368);
#2746=AXIS2_PLACEMENT_3D('',#7340,#3370,#3371);
#2747=AXIS2_PLACEMENT_3D('',#7342,#3372,#3373);
#2748=AXIS2_PLACEMENT_3D('',#7344,#3374,#3375);
#2749=AXIS2_PLACEMENT_3D('',#7345,#3376,#3377);
#2750=AXIS2_PLACEMENT_3D('',#7346,#3378,#3379);
#2751=AXIS2_PLACEMENT_3D('',#7348,#3380,#3381);
#2752=AXIS2_PLACEMENT_3D('',#7350,#3382,#3383);
#2753=AXIS2_PLACEMENT_3D('',#7351,#3384,#3385);
#2754=AXIS2_PLACEMENT_3D('',#7352,#3386,#3387);
#2755=AXIS2_PLACEMENT_3D('',#7354,#3389,#3390);
#2756=AXIS2_PLACEMENT_3D('',#7356,#3392,#3393);
#2757=AXIS2_PLACEMENT_3D('',#7358,#3394,#3395);
#2758=AXIS2_PLACEMENT_3D('',#7360,#3396,#3397);
#2759=AXIS2_PLACEMENT_3D('',#7361,#3398,#3399);
#2760=AXIS2_PLACEMENT_3D('',#7362,#3400,#3401);
#2761=AXIS2_PLACEMENT_3D('',#7364,#3402,#3403);
#2762=AXIS2_PLACEMENT_3D('',#7366,#3404,#3405);
#2763=AXIS2_PLACEMENT_3D('',#7367,#3406,#3407);
#2764=AXIS2_PLACEMENT_3D('',#7368,#3408,#3409);
#2765=AXIS2_PLACEMENT_3D('',#7370,#3411,#3412);
#2766=AXIS2_PLACEMENT_3D('',#7372,#3414,#3415);
#2767=AXIS2_PLACEMENT_3D('',#7374,#3416,#3417);
#2768=AXIS2_PLACEMENT_3D('',#7376,#3418,#3419);
#2769=AXIS2_PLACEMENT_3D('',#7377,#3420,#3421);
#2770=AXIS2_PLACEMENT_3D('',#7378,#3422,#3423);
#2771=AXIS2_PLACEMENT_3D('',#7380,#3424,#3425);
#2772=AXIS2_PLACEMENT_3D('',#7382,#3426,#3427);
#2773=AXIS2_PLACEMENT_3D('',#7383,#3428,#3429);
#2774=AXIS2_PLACEMENT_3D('',#7384,#3430,#3431);
#2775=AXIS2_PLACEMENT_3D('',#7386,#3433,#3434);
#3148=DIRECTION('axis',(0.,0.,1.));
#3149=DIRECTION('refdir',(1.,0.,0.));
#3150=DIRECTION('center_axis',(0.,-1.,0.));
#3151=DIRECTION('ref_axis',(1.22464679914735E-16,0.,1.));
#3152=DIRECTION('center_axis',(0.,0.,1.));
#3153=DIRECTION('ref_axis',(1.,0.,0.));
#3154=DIRECTION('center_axis',(0.,1.,0.));
#3155=DIRECTION('ref_axis',(1.22464679914735E-16,0.,1.));
#3156=DIRECTION('center_axis',(-4.91504984860095E-16,0.,-1.));
#3157=DIRECTION('ref_axis',(-1.,0.,4.91504984860095E-16));
#3158=DIRECTION('center_axis',(0.,-1.,0.));
#3159=DIRECTION('ref_axis',(0.,0.,-1.));
#3160=DIRECTION('center_axis',(-3.37307342551046E-16,0.,-1.));
#3161=DIRECTION('ref_axis',(-1.,0.,3.37307342551046E-16));
#3162=DIRECTION('center_axis',(0.,1.,0.));
#3163=DIRECTION('ref_axis',(0.,0.,-1.));
#3164=DIRECTION('center_axis',(0.,0.,1.));
#3165=DIRECTION('ref_axis',(1.,0.,0.));
#3166=DIRECTION('center_axis',(-3.46944695195361E-16,0.,-1.));
#3167=DIRECTION('ref_axis',(-1.,0.,3.46944695195361E-16));
#3168=DIRECTION('',(3.46944695195361E-16,0.,1.));
#3169=DIRECTION('center_axis',(3.46944695195361E-16,0.,1.));
#3170=DIRECTION('ref_axis',(1.,0.,-3.46944695195361E-16));
#3171=DIRECTION('',(-3.46944695195361E-16,0.,-1.));
#3172=DIRECTION('center_axis',(0.,-1.,0.));
#3173=DIRECTION('ref_axis',(1.22464679914735E-16,0.,1.));
#3174=DIRECTION('center_axis',(0.,0.,1.));
#3175=DIRECTION('ref_axis',(1.,0.,0.));
#3176=DIRECTION('center_axis',(0.,1.,0.));
#3177=DIRECTION('ref_axis',(1.22464679914735E-16,0.,1.));
#3178=DIRECTION('center_axis',(-4.91504984860095E-16,0.,-1.));
#3179=DIRECTION('ref_axis',(-1.,0.,4.91504984860095E-16));
#3180=DIRECTION('center_axis',(0.,-1.,0.));
#3181=DIRECTION('ref_axis',(0.,0.,-1.));
#3182=DIRECTION('center_axis',(-3.37307342551046E-16,0.,-1.));
#3183=DIRECTION('ref_axis',(-1.,0.,3.37307342551046E-16));
#3184=DIRECTION('center_axis',(0.,1.,0.));
#3185=DIRECTION('ref_axis',(0.,0.,-1.));
#3186=DIRECTION('center_axis',(0.,0.,1.));
#3187=DIRECTION('ref_axis',(1.,0.,0.));
#3188=DIRECTION('center_axis',(-3.46944695195361E-16,0.,-1.));
#3189=DIRECTION('ref_axis',(-1.,0.,3.46944695195361E-16));
#3190=DIRECTION('',(3.46944695195361E-16,0.,1.));
#3191=DIRECTION('center_axis',(3.46944695195361E-16,0.,1.));
#3192=DIRECTION('ref_axis',(1.,0.,-3.46944695195361E-16));
#3193=DIRECTION('',(-3.46944695195361E-16,0.,-1.));
#3194=DIRECTION('center_axis',(0.,-1.,0.));
#3195=DIRECTION('ref_axis',(1.22464679914735E-16,0.,1.));
#3196=DIRECTION('center_axis',(0.,0.,1.));
#3197=DIRECTION('ref_axis',(1.,0.,0.));
#3198=DIRECTION('center_axis',(0.,1.,0.));
#3199=DIRECTION('ref_axis',(1.22464679914735E-16,0.,1.));
#3200=DIRECTION('center_axis',(-4.91504984860095E-16,0.,-1.));
#3201=DIRECTION('ref_axis',(-1.,0.,4.91504984860095E-16));
#3202=DIRECTION('center_axis',(0.,-1.,0.));
#3203=DIRECTION('ref_axis',(0.,0.,-1.));
#3204=DIRECTION('center_axis',(-3.37307342551046E-16,0.,-1.));
#3205=DIRECTION('ref_axis',(-1.,0.,3.37307342551046E-16));
#3206=DIRECTION('center_axis',(0.,1.,0.));
#3207=DIRECTION('ref_axis',(0.,0.,-1.));
#3208=DIRECTION('center_axis',(0.,0.,1.));
#3209=DIRECTION('ref_axis',(1.,0.,0.));
#3210=DIRECTION('center_axis',(-3.46944695195361E-16,0.,-1.));
#3211=DIRECTION('ref_axis',(-1.,0.,3.46944695195361E-16));
#3212=DIRECTION('',(3.46944695195361E-16,0.,1.));
#3213=DIRECTION('center_axis',(3.46944695195361E-16,0.,1.));
#3214=DIRECTION('ref_axis',(1.,0.,-3.46944695195361E-16));
#3215=DIRECTION('',(-3.46944695195361E-16,0.,-1.));
#3216=DIRECTION('center_axis',(0.,-1.,0.));
#3217=DIRECTION('ref_axis',(1.22464679914735E-16,0.,1.));
#3218=DIRECTION('center_axis',(0.,0.,1.));
#3219=DIRECTION('ref_axis',(1.,0.,0.));
#3220=DIRECTION('center_axis',(0.,1.,0.));
#3221=DIRECTION('ref_axis',(1.22464679914735E-16,0.,1.));
#3222=DIRECTION('center_axis',(-4.91504984860095E-16,0.,-1.));
#3223=DIRECTION('ref_axis',(-1.,0.,4.91504984860095E-16));
#3224=DIRECTION('center_axis',(0.,-1.,0.));
#3225=DIRECTION('ref_axis',(0.,0.,-1.));
#3226=DIRECTION('center_axis',(-3.37307342551046E-16,0.,-1.));
#3227=DIRECTION('ref_axis',(-1.,0.,3.37307342551046E-16));
#3228=DIRECTION('center_axis',(0.,1.,0.));
#3229=DIRECTION('ref_axis',(0.,0.,-1.));
#3230=DIRECTION('center_axis',(0.,0.,1.));
#3231=DIRECTION('ref_axis',(1.,0.,0.));
#3232=DIRECTION('center_axis',(-3.46944695195361E-16,0.,-1.));
#3233=DIRECTION('ref_axis',(-1.,0.,3.46944695195361E-16));
#3234=DIRECTION('',(3.46944695195361E-16,0.,1.));
#3235=DIRECTION('center_axis',(3.46944695195361E-16,0.,1.));
#3236=DIRECTION('ref_axis',(1.,0.,-3.46944695195361E-16));
#3237=DIRECTION('',(-3.46944695195361E-16,0.,-1.));
#3238=DIRECTION('center_axis',(0.,-1.,0.));
#3239=DIRECTION('ref_axis',(1.22464679914735E-16,0.,1.));
#3240=DIRECTION('center_axis',(0.,0.,1.));
#3241=DIRECTION('ref_axis',(1.,0.,0.));
#3242=DIRECTION('center_axis',(0.,1.,0.));
#3243=DIRECTION('ref_axis',(1.22464679914735E-16,0.,1.));
#3244=DIRECTION('center_axis',(-4.91504984860095E-16,0.,-1.));
#3245=DIRECTION('ref_axis',(-1.,0.,4.91504984860095E-16));
#3246=DIRECTION('center_axis',(0.,-1.,0.));
#3247=DIRECTION('ref_axis',(0.,0.,-1.));
#3248=DIRECTION('center_axis',(-3.37307342551046E-16,0.,-1.));
#3249=DIRECTION('ref_axis',(-1.,0.,3.37307342551046E-16));
#3250=DIRECTION('center_axis',(0.,1.,0.));
#3251=DIRECTION('ref_axis',(0.,0.,-1.));
#3252=DIRECTION('center_axis',(0.,0.,1.));
#3253=DIRECTION('ref_axis',(1.,0.,0.));
#3254=DIRECTION('center_axis',(-3.46944695195361E-16,0.,-1.));
#3255=DIRECTION('ref_axis',(-1.,0.,3.46944695195361E-16));
#3256=DIRECTION('',(3.46944695195361E-16,0.,1.));
#3257=DIRECTION('center_axis',(3.46944695195361E-16,0.,1.));
#3258=DIRECTION('ref_axis',(1.,0.,-3.46944695195361E-16));
#3259=DIRECTION('',(-3.46944695195361E-16,0.,-1.));
#3260=DIRECTION('center_axis',(0.,-1.,0.));
#3261=DIRECTION('ref_axis',(1.22464679914735E-16,0.,1.));
#3262=DIRECTION('center_axis',(0.,0.,1.));
#3263=DIRECTION('ref_axis',(1.,0.,0.));
#3264=DIRECTION('center_axis',(0.,1.,0.));
#3265=DIRECTION('ref_axis',(1.22464679914735E-16,0.,1.));
#3266=DIRECTION('center_axis',(-4.91504984860095E-16,0.,-1.));
#3267=DIRECTION('ref_axis',(-1.,0.,4.91504984860095E-16));
#3268=DIRECTION('center_axis',(0.,-1.,0.));
#3269=DIRECTION('ref_axis',(0.,0.,-1.));
#3270=DIRECTION('center_axis',(-3.37307342551046E-16,0.,-1.));
#3271=DIRECTION('ref_axis',(-1.,0.,3.37307342551046E-16));
#3272=DIRECTION('center_axis',(0.,1.,0.));
#3273=DIRECTION('ref_axis',(0.,0.,-1.));
#3274=DIRECTION('center_axis',(0.,0.,1.));
#3275=DIRECTION('ref_axis',(1.,0.,0.));
#3276=DIRECTION('center_axis',(-3.46944695195361E-16,0.,-1.));
#3277=DIRECTION('ref_axis',(-1.,0.,3.46944695195361E-16));
#3278=DIRECTION('',(3.46944695195361E-16,0.,1.));
#3279=DIRECTION('center_axis',(3.46944695195361E-16,0.,1.));
#3280=DIRECTION('ref_axis',(1.,0.,-3.46944695195361E-16));
#3281=DIRECTION('',(-3.46944695195361E-16,0.,-1.));
#3282=DIRECTION('center_axis',(0.,-1.,0.));
#3283=DIRECTION('ref_axis',(1.22464679914735E-16,0.,1.));
#3284=DIRECTION('center_axis',(0.,0.,1.));
#3285=DIRECTION('ref_axis',(1.,0.,0.));
#3286=DIRECTION('center_axis',(0.,1.,0.));
#3287=DIRECTION('ref_axis',(1.22464679914735E-16,0.,1.));
#3288=DIRECTION('center_axis',(-4.91504984860095E-16,0.,-1.));
#3289=DIRECTION('ref_axis',(-1.,0.,4.91504984860095E-16));
#3290=DIRECTION('center_axis',(0.,-1.,0.));
#3291=DIRECTION('ref_axis',(0.,0.,-1.));
#3292=DIRECTION('center_axis',(-3.37307342551046E-16,0.,-1.));
#3293=DIRECTION('ref_axis',(-1.,0.,3.37307342551046E-16));
#3294=DIRECTION('center_axis',(0.,1.,0.));
#3295=DIRECTION('ref_axis',(0.,0.,-1.));
#3296=DIRECTION('center_axis',(0.,0.,1.));
#3297=DIRECTION('ref_axis',(1.,0.,0.));
#3298=DIRECTION('center_axis',(-3.46944695195361E-16,0.,-1.));
#3299=DIRECTION('ref_axis',(-1.,0.,3.46944695195361E-16));
#3300=DIRECTION('',(3.46944695195361E-16,0.,1.));
#3301=DIRECTION('center_axis',(3.46944695195361E-16,0.,1.));
#3302=DIRECTION('ref_axis',(1.,0.,-3.46944695195361E-16));
#3303=DIRECTION('',(-3.46944695195361E-16,0.,-1.));
#3304=DIRECTION('center_axis',(0.,-1.,0.));
#3305=DIRECTION('ref_axis',(1.22464679914735E-16,0.,1.));
#3306=DIRECTION('center_axis',(0.,0.,1.));
#3307=DIRECTION('ref_axis',(1.,0.,0.));
#3308=DIRECTION('center_axis',(0.,1.,0.));
#3309=DIRECTION('ref_axis',(1.22464679914735E-16,0.,1.));
#3310=DIRECTION('center_axis',(-4.91504984860095E-16,0.,-1.));
#3311=DIRECTION('ref_axis',(-1.,0.,4.91504984860095E-16));
#3312=DIRECTION('center_axis',(0.,-1.,0.));
#3313=DIRECTION('ref_axis',(0.,0.,-1.));
#3314=DIRECTION('center_axis',(-3.37307342551046E-16,0.,-1.));
#3315=DIRECTION('ref_axis',(-1.,0.,3.37307342551046E-16));
#3316=DIRECTION('center_axis',(0.,1.,0.));
#3317=DIRECTION('ref_axis',(0.,0.,-1.));
#3318=DIRECTION('center_axis',(0.,0.,1.));
#3319=DIRECTION('ref_axis',(1.,0.,0.));
#3320=DIRECTION('center_axis',(-3.46944695195361E-16,0.,-1.));
#3321=DIRECTION('ref_axis',(-1.,0.,3.46944695195361E-16));
#3322=DIRECTION('',(3.46944695195361E-16,0.,1.));
#3323=DIRECTION('center_axis',(3.46944695195361E-16,0.,1.));
#3324=DIRECTION('ref_axis',(1.,0.,-3.46944695195361E-16));
#3325=DIRECTION('',(-3.46944695195361E-16,0.,-1.));
#3326=DIRECTION('center_axis',(0.,-1.,0.));
#3327=DIRECTION('ref_axis',(1.22464679914735E-16,0.,1.));
#3328=DIRECTION('center_axis',(0.,0.,1.));
#3329=DIRECTION('ref_axis',(1.,0.,0.));
#3330=DIRECTION('center_axis',(0.,1.,0.));
#3331=DIRECTION('ref_axis',(1.22464679914735E-16,0.,1.));
#3332=DIRECTION('center_axis',(-4.91504984860095E-16,0.,-1.));
#3333=DIRECTION('ref_axis',(-1.,0.,4.91504984860095E-16));
#3334=DIRECTION('center_axis',(0.,-1.,0.));
#3335=DIRECTION('ref_axis',(0.,0.,-1.));
#3336=DIRECTION('center_axis',(-3.37307342551046E-16,0.,-1.));
#3337=DIRECTION('ref_axis',(-1.,0.,3.37307342551046E-16));
#3338=DIRECTION('center_axis',(0.,1.,0.));
#3339=DIRECTION('ref_axis',(0.,0.,-1.));
#3340=DIRECTION('center_axis',(0.,0.,1.));
#3341=DIRECTION('ref_axis',(1.,0.,0.));
#3342=DIRECTION('center_axis',(-3.46944695195361E-16,0.,-1.));
#3343=DIRECTION('ref_axis',(-1.,0.,3.46944695195361E-16));
#3344=DIRECTION('',(3.46944695195361E-16,0.,1.));
#3345=DIRECTION('center_axis',(3.46944695195361E-16,0.,1.));
#3346=DIRECTION('ref_axis',(1.,0.,-3.46944695195361E-16));
#3347=DIRECTION('',(-3.46944695195361E-16,0.,-1.));
#3348=DIRECTION('center_axis',(0.,-1.,0.));
#3349=DIRECTION('ref_axis',(1.22464679914735E-16,0.,1.));
#3350=DIRECTION('center_axis',(0.,0.,1.));
#3351=DIRECTION('ref_axis',(1.,0.,0.));
#3352=DIRECTION('center_axis',(0.,1.,0.));
#3353=DIRECTION('ref_axis',(1.22464679914735E-16,0.,1.));
#3354=DIRECTION('center_axis',(-4.91504984860095E-16,0.,-1.));
#3355=DIRECTION('ref_axis',(-1.,0.,4.91504984860095E-16));
#3356=DIRECTION('center_axis',(0.,-1.,0.));
#3357=DIRECTION('ref_axis',(0.,0.,-1.));
#3358=DIRECTION('center_axis',(-3.37307342551046E-16,0.,-1.));
#3359=DIRECTION('ref_axis',(-1.,0.,3.37307342551046E-16));
#3360=DIRECTION('center_axis',(0.,1.,0.));
#3361=DIRECTION('ref_axis',(0.,0.,-1.));
#3362=DIRECTION('center_axis',(0.,0.,1.));
#3363=DIRECTION('ref_axis',(1.,0.,0.));
#3364=DIRECTION('center_axis',(-3.46944695195361E-16,0.,-1.));
#3365=DIRECTION('ref_axis',(-1.,0.,3.46944695195361E-16));
#3366=DIRECTION('',(3.46944695195361E-16,0.,1.));
#3367=DIRECTION('center_axis',(3.46944695195361E-16,0.,1.));
#3368=DIRECTION('ref_axis',(1.,0.,-3.46944695195361E-16));
#3369=DIRECTION('',(-3.46944695195361E-16,0.,-1.));
#3370=DIRECTION('center_axis',(0.,-1.,0.));
#3371=DIRECTION('ref_axis',(1.22464679914735E-16,0.,1.));
#3372=DIRECTION('center_axis',(0.,0.,1.));
#3373=DIRECTION('ref_axis',(1.,0.,0.));
#3374=DIRECTION('center_axis',(0.,1.,0.));
#3375=DIRECTION('ref_axis',(1.22464679914735E-16,0.,1.));
#3376=DIRECTION('center_axis',(-4.91504984860095E-16,0.,-1.));
#3377=DIRECTION('ref_axis',(-1.,0.,4.91504984860095E-16));
#3378=DIRECTION('center_axis',(0.,-1.,0.));
#3379=DIRECTION('ref_axis',(0.,0.,-1.));
#3380=DIRECTION('center_axis',(-3.37307342551046E-16,0.,-1.));
#3381=DIRECTION('ref_axis',(-1.,0.,3.37307342551046E-16));
#3382=DIRECTION('center_axis',(0.,1.,0.));
#3383=DIRECTION('ref_axis',(0.,0.,-1.));
#3384=DIRECTION('center_axis',(0.,0.,1.));
#3385=DIRECTION('ref_axis',(1.,0.,0.));
#3386=DIRECTION('center_axis',(-3.46944695195361E-16,0.,-1.));
#3387=DIRECTION('ref_axis',(-1.,0.,3.46944695195361E-16));
#3388=DIRECTION('',(3.46944695195361E-16,0.,1.));
#3389=DIRECTION('center_axis',(3.46944695195361E-16,0.,1.));
#3390=DIRECTION('ref_axis',(1.,0.,-3.46944695195361E-16));
#3391=DIRECTION('',(-3.46944695195361E-16,0.,-1.));
#3392=DIRECTION('center_axis',(0.,-1.,0.));
#3393=DIRECTION('ref_axis',(1.22464679914735E-16,0.,1.));
#3394=DIRECTION('center_axis',(0.,0.,1.));
#3395=DIRECTION('ref_axis',(1.,0.,0.));
#3396=DIRECTION('center_axis',(0.,1.,0.));
#3397=DIRECTION('ref_axis',(1.22464679914735E-16,0.,1.));
#3398=DIRECTION('center_axis',(-4.91504984860095E-16,0.,-1.));
#3399=DIRECTION('ref_axis',(-1.,0.,4.91504984860095E-16));
#3400=DIRECTION('center_axis',(0.,-1.,0.));
#3401=DIRECTION('ref_axis',(0.,0.,-1.));
#3402=DIRECTION('center_axis',(-3.37307342551046E-16,0.,-1.));
#3403=DIRECTION('ref_axis',(-1.,0.,3.37307342551046E-16));
#3404=DIRECTION('center_axis',(0.,1.,0.));
#3405=DIRECTION('ref_axis',(0.,0.,-1.));
#3406=DIRECTION('center_axis',(0.,0.,1.));
#3407=DIRECTION('ref_axis',(1.,0.,0.));
#3408=DIRECTION('center_axis',(-3.46944695195361E-16,0.,-1.));
#3409=DIRECTION('ref_axis',(-1.,0.,3.46944695195361E-16));
#3410=DIRECTION('',(3.46944695195361E-16,0.,1.));
#3411=DIRECTION('center_axis',(3.46944695195361E-16,0.,1.));
#3412=DIRECTION('ref_axis',(1.,0.,-3.46944695195361E-16));
#3413=DIRECTION('',(-3.46944695195361E-16,0.,-1.));
#3414=DIRECTION('center_axis',(0.,-1.,0.));
#3415=DIRECTION('ref_axis',(1.22464679914735E-16,0.,1.));
#3416=DIRECTION('center_axis',(0.,0.,1.));
#3417=DIRECTION('ref_axis',(1.,0.,0.));
#3418=DIRECTION('center_axis',(0.,1.,0.));
#3419=DIRECTION('ref_axis',(1.22464679914735E-16,0.,1.));
#3420=DIRECTION('center_axis',(-4.91504984860095E-16,0.,-1.));
#3421=DIRECTION('ref_axis',(-1.,0.,4.91504984860095E-16));
#3422=DIRECTION('center_axis',(0.,-1.,0.));
#3423=DIRECTION('ref_axis',(0.,0.,-1.));
#3424=DIRECTION('center_axis',(-3.37307342551046E-16,0.,-1.));
#3425=DIRECTION('ref_axis',(-1.,0.,3.37307342551046E-16));
#3426=DIRECTION('center_axis',(0.,1.,0.));
#3427=DIRECTION('ref_axis',(0.,0.,-1.));
#3428=DIRECTION('center_axis',(0.,0.,1.));
#3429=DIRECTION('ref_axis',(1.,0.,0.));
#3430=DIRECTION('center_axis',(-3.46944695195361E-16,0.,-1.));
#3431=DIRECTION('ref_axis',(-1.,0.,3.46944695195361E-16));
#3432=DIRECTION('',(3.46944695195361E-16,0.,1.));
#3433=DIRECTION('center_axis',(3.46944695195361E-16,0.,1.));
#3434=DIRECTION('ref_axis',(1.,0.,-3.46944695195361E-16));
#3435=DIRECTION('',(-3.46944695195361E-16,0.,-1.));
#7179=CARTESIAN_POINT('',(0.,0.,0.));
#7180=CARTESIAN_POINT('Origin',(0.,43.,2.5));
#7181=CARTESIAN_POINT('',(-8.,43.,2.5));
#7182=CARTESIAN_POINT('Origin',(-9.,43.,2.5));
#7183=CARTESIAN_POINT('',(8.00000000000001,43.,2.5));
#7184=CARTESIAN_POINT('Origin',(0.,43.,2.5));
#7185=CARTESIAN_POINT('Origin',(9.00000000000001,43.,2.5));
#7186=CARTESIAN_POINT('Origin',(-1.73472347597681E-15,43.,-2.5));
#7187=CARTESIAN_POINT('',(8.,43.,-2.5));
#7188=CARTESIAN_POINT('Origin',(9.,43.,-2.5));
#7189=CARTESIAN_POINT('',(-8.,43.,-2.5));
#7190=CARTESIAN_POINT('Origin',(-1.73472347597681E-15,43.,-2.5));
#7191=CARTESIAN_POINT('Origin',(-9.,43.,-2.5));
#7192=CARTESIAN_POINT('Origin',(-9.,43.,2.5));
#7193=CARTESIAN_POINT('',(-8.,43.,2.5));
#7194=CARTESIAN_POINT('Origin',(9.,43.,-2.5));
#7195=CARTESIAN_POINT('',(8.,43.,-2.5));
#7196=CARTESIAN_POINT('Origin',(0.,40.8,2.5));
#7197=CARTESIAN_POINT('',(-8.,40.8,2.5));
#7198=CARTESIAN_POINT('Origin',(-9.,40.8,2.5));
#7199=CARTESIAN_POINT('',(8.00000000000001,40.8,2.5));
#7200=CARTESIAN_POINT('Origin',(0.,40.8,2.5));
#7201=CARTESIAN_POINT('Origin',(9.00000000000001,40.8,2.5));
#7202=CARTESIAN_POINT('Origin',(-1.73472347597681E-15,40.8,-2.5));
#7203=CARTESIAN_POINT('',(8.,40.8,-2.5));
#7204=CARTESIAN_POINT('Origin',(9.,40.8,-2.5));
#7205=CARTESIAN_POINT('',(-8.,40.8,-2.5));
#7206=CARTESIAN_POINT('Origin',(-1.73472347597681E-15,40.8,-2.5));
#7207=CARTESIAN_POINT('Origin',(-9.,40.8,-2.5));
#7208=CARTESIAN_POINT('Origin',(-9.,40.8,2.5));
#7209=CARTESIAN_POINT('',(-8.,40.8,2.5));
#7210=CARTESIAN_POINT('Origin',(9.,40.8,-2.5));
#7211=CARTESIAN_POINT('',(8.,40.8,-2.5));
#7212=CARTESIAN_POINT('Origin',(0.,38.6,2.5));
#7213=CARTESIAN_POINT('',(-8.,38.6,2.5));
#7214=CARTESIAN_POINT('Origin',(-9.,38.6,2.5));
#7215=CARTESIAN_POINT('',(8.00000000000001,38.6,2.5));
#7216=CARTESIAN_POINT('Origin',(0.,38.6,2.5));
#7217=CARTESIAN_POINT('Origin',(9.00000000000001,38.6,2.5));
#7218=CARTESIAN_POINT('Origin',(-1.73472347597681E-15,38.6,-2.5));
#7219=CARTESIAN_POINT('',(8.,38.6,-2.5));
#7220=CARTESIAN_POINT('Origin',(9.,38.6,-2.5));
#7221=CARTESIAN_POINT('',(-8.,38.6,-2.5));
#7222=CARTESIAN_POINT('Origin',(-1.73472347597681E-15,38.6,-2.5));
#7223=CARTESIAN_POINT('Origin',(-9.,38.6,-2.5));
#7224=CARTESIAN_POINT('Origin',(-9.,38.6,2.5));
#7225=CARTESIAN_POINT('',(-8.,38.6,2.5));
#7226=CARTESIAN_POINT('Origin',(9.,38.6,-2.5));
#7227=CARTESIAN_POINT('',(8.,38.6,-2.5));
#7228=CARTESIAN_POINT('Origin',(0.,36.4,2.5));
#7229=CARTESIAN_POINT('',(-8.,36.4,2.5));
#7230=CARTESIAN_POINT('Origin',(-9.,36.4,2.5));
#7231=CARTESIAN_POINT('',(8.00000000000001,36.4,2.5));
#7232=CARTESIAN_POINT('Origin',(0.,36.4,2.5));
#7233=CARTESIAN_POINT('Origin',(9.00000000000001,36.4,2.5));
#7234=CARTESIAN_POINT('Origin',(-1.73472347597681E-15,36.4,-2.5));
#7235=CARTESIAN_POINT('',(8.,36.4,-2.5));
#7236=CARTESIAN_POINT('Origin',(9.,36.4,-2.5));
#7237=CARTESIAN_POINT('',(-8.,36.4,-2.5));
#7238=CARTESIAN_POINT('Origin',(-1.73472347597681E-15,36.4,-2.5));
#7239=CARTESIAN_POINT('Origin',(-9.,36.4,-2.5));
#7240=CARTESIAN_POINT('Origin',(-9.,36.4,2.5));
#7241=CARTESIAN_POINT('',(-8.,36.4,2.5));
#7242=CARTESIAN_POINT('Origin',(9.,36.4,-2.5));
#7243=CARTESIAN_POINT('',(8.,36.4,-2.5));
#7244=CARTESIAN_POINT('Origin',(0.,34.2,2.5));
#7245=CARTESIAN_POINT('',(-8.,34.2,2.5));
#7246=CARTESIAN_POINT('Origin',(-9.,34.2,2.5));
#7247=CARTESIAN_POINT('',(8.00000000000001,34.2,2.5));
#7248=CARTESIAN_POINT('Origin',(0.,34.2,2.5));
#7249=CARTESIAN_POINT('Origin',(9.00000000000001,34.2,2.5));
#7250=CARTESIAN_POINT('Origin',(-1.73472347597681E-15,34.2,-2.5));
#7251=CARTESIAN_POINT('',(8.,34.2,-2.5));
#7252=CARTESIAN_POINT('Origin',(9.,34.2,-2.5));
#7253=CARTESIAN_POINT('',(-8.,34.2,-2.5));
#7254=CARTESIAN_POINT('Origin',(-1.73472347597681E-15,34.2,-2.5));
#7255=CARTESIAN_POINT('Origin',(-9.,34.2,-2.5));
#7256=CARTESIAN_POINT('Origin',(-9.,34.2,2.5));
#7257=CARTESIAN_POINT('',(-8.,34.2,2.5));
#7258=CARTESIAN_POINT('Origin',(9.,34.2,-2.5));
#7259=CARTESIAN_POINT('',(8.,34.2,-2.5));
#7260=CARTESIAN_POINT('Origin',(0.,32.,2.5));
#7261=CARTESIAN_POINT('',(-8.,32.,2.5));
#7262=CARTESIAN_POINT('Origin',(-9.,32.,2.5));
#7263=CARTESIAN_POINT('',(8.00000000000001,32.,2.5));
#7264=CARTESIAN_POINT('Origin',(0.,32.,2.5));
#7265=CARTESIAN_POINT('Origin',(9.00000000000001,32.,2.5));
#7266=CARTESIAN_POINT('Origin',(-1.73472347597681E-15,32.,-2.5));
#7267=CARTESIAN_POINT('',(8.,32.,-2.5));
#7268=CARTESIAN_POINT('Origin',(9.,32.,-2.5));
#7269=CARTESIAN_POINT('',(-8.,32.,-2.5));
#7270=CARTESIAN_POINT('Origin',(-1.73472347597681E-15,32.,-2.5));
#7271=CARTESIAN_POINT('Origin',(-9.,32.,-2.5));
#7272=CARTESIAN_POINT('Origin',(-9.,32.,2.5));
#7273=CARTESIAN_POINT('',(-8.,32.,2.5));
#7274=CARTESIAN_POINT('Origin',(9.,32.,-2.5));
#7275=CARTESIAN_POINT('',(8.,32.,-2.5));
#7276=CARTESIAN_POINT('Origin',(0.,29.8,2.5));
#7277=CARTESIAN_POINT('',(-8.,29.8,2.5));
#7278=CARTESIAN_POINT('Origin',(-9.,29.8,2.5));
#7279=CARTESIAN_POINT('',(8.00000000000001,29.8,2.5));
#7280=CARTESIAN_POINT('Origin',(0.,29.8,2.5));
#7281=CARTESIAN_POINT('Origin',(9.00000000000001,29.8,2.5));
#7282=CARTESIAN_POINT('Origin',(-1.73472347597681E-15,29.8,-2.5));
#7283=CARTESIAN_POINT('',(8.,29.8,-2.5));
#7284=CARTESIAN_POINT('Origin',(9.,29.8,-2.5));
#7285=CARTESIAN_POINT('',(-8.,29.8,-2.5));
#7286=CARTESIAN_POINT('Origin',(-1.73472347597681E-15,29.8,-2.5));
#7287=CARTESIAN_POINT('Origin',(-9.,29.8,-2.5));
#7288=CARTESIAN_POINT('Origin',(-9.,29.8,2.5));
#7289=CARTESIAN_POINT('',(-8.,29.8,2.5));
#7290=CARTESIAN_POINT('Origin',(9.,29.8,-2.5));
#7291=CARTESIAN_POINT('',(8.,29.8,-2.5));
#7292=CARTESIAN_POINT('Origin',(0.,27.6,2.5));
#7293=CARTESIAN_POINT('',(-8.,27.6,2.5));
#7294=CARTESIAN_POINT('Origin',(-9.,27.6,2.5));
#7295=CARTESIAN_POINT('',(8.00000000000001,27.6,2.5));
#7296=CARTESIAN_POINT('Origin',(0.,27.6,2.5));
#7297=CARTESIAN_POINT('Origin',(9.00000000000001,27.6,2.5));
#7298=CARTESIAN_POINT('Origin',(-1.73472347597681E-15,27.6,-2.5));
#7299=CARTESIAN_POINT('',(8.,27.6,-2.5));
#7300=CARTESIAN_POINT('Origin',(9.,27.6,-2.5));
#7301=CARTESIAN_POINT('',(-8.,27.6,-2.5));
#7302=CARTESIAN_POINT('Origin',(-1.73472347597681E-15,27.6,-2.5));
#7303=CARTESIAN_POINT('Origin',(-9.,27.6,-2.5));
#7304=CARTESIAN_POINT('Origin',(-9.,27.6,2.5));
#7305=CARTESIAN_POINT('',(-8.,27.6,2.5));
#7306=CARTESIAN_POINT('Origin',(9.,27.6,-2.5));
#7307=CARTESIAN_POINT('',(8.,27.6,-2.5));
#7308=CARTESIAN_POINT('Origin',(0.,25.4,2.5));
#7309=CARTESIAN_POINT('',(-8.,25.4,2.5));
#7310=CARTESIAN_POINT('Origin',(-9.,25.4,2.5));
#7311=CARTESIAN_POINT('',(8.00000000000001,25.4,2.5));
#7312=CARTESIAN_POINT('Origin',(0.,25.4,2.5));
#7313=CARTESIAN_POINT('Origin',(9.00000000000001,25.4,2.5));
#7314=CARTESIAN_POINT('Origin',(-1.73472347597681E-15,25.4,-2.5));
#7315=CARTESIAN_POINT('',(8.,25.4,-2.5));
#7316=CARTESIAN_POINT('Origin',(9.,25.4,-2.5));
#7317=CARTESIAN_POINT('',(-8.,25.4,-2.5));
#7318=CARTESIAN_POINT('Origin',(-1.73472347597681E-15,25.4,-2.5));
#7319=CARTESIAN_POINT('Origin',(-9.,25.4,-2.5));
#7320=CARTESIAN_POINT('Origin',(-9.,25.4,2.5));
#7321=CARTESIAN_POINT('',(-8.,25.4,2.5));
#7322=CARTESIAN_POINT('Origin',(9.,25.4,-2.5));
#7323=CARTESIAN_POINT('',(8.,25.4,-2.5));
#7324=CARTESIAN_POINT('Origin',(0.,23.2,2.5));
#7325=CARTESIAN_POINT('',(-8.,23.2,2.5));
#7326=CARTESIAN_POINT('Origin',(-9.,23.2,2.5));
#7327=CARTESIAN_POINT('',(8.00000000000001,23.2,2.5));
#7328=CARTESIAN_POINT('Origin',(0.,23.2,2.5));
#7329=CARTESIAN_POINT('Origin',(9.00000000000001,23.2,2.5));
#7330=CARTESIAN_POINT('Origin',(-1.73472347597681E-15,23.2,-2.5));
#7331=CARTESIAN_POINT('',(8.,23.2,-2.5));
#7332=CARTESIAN_POINT('Origin',(9.,23.2,-2.5));
#7333=CARTESIAN_POINT('',(-8.,23.2,-2.5));
#7334=CARTESIAN_POINT('Origin',(-1.73472347597681E-15,23.2,-2.5));
#7335=CARTESIAN_POINT('Origin',(-9.,23.2,-2.5));
#7336=CARTESIAN_POINT('Origin',(-9.,23.2,2.5));
#7337=CARTESIAN_POINT('',(-8.,23.2,2.5));
#7338=CARTESIAN_POINT('Origin',(9.,23.2,-2.5));
#7339=CARTESIAN_POINT('',(8.,23.2,-2.5));
#7340=CARTESIAN_POINT('Origin',(0.,21.,2.5));
#7341=CARTESIAN_POINT('',(-8.,21.,2.5));
#7342=CARTESIAN_POINT('Origin',(-9.,21.,2.5));
#7343=CARTESIAN_POINT('',(8.00000000000001,21.,2.5));
#7344=CARTESIAN_POINT('Origin',(0.,21.,2.5));
#7345=CARTESIAN_POINT('Origin',(9.00000000000001,21.,2.5));
#7346=CARTESIAN_POINT('Origin',(-1.73472347597681E-15,21.,-2.5));
#7347=CARTESIAN_POINT('',(8.,21.,-2.5));
#7348=CARTESIAN_POINT('Origin',(9.,21.,-2.5));
#7349=CARTESIAN_POINT('',(-8.,21.,-2.5));
#7350=CARTESIAN_POINT('Origin',(-1.73472347597681E-15,21.,-2.5));
#7351=CARTESIAN_POINT('Origin',(-9.,21.,-2.5));
#7352=CARTESIAN_POINT('Origin',(-9.,21.,2.5));
#7353=CARTESIAN_POINT('',(-8.,21.,2.5));
#7354=CARTESIAN_POINT('Origin',(9.,21.,-2.5));
#7355=CARTESIAN_POINT('',(8.,21.,-2.5));
#7356=CARTESIAN_POINT('Origin',(0.,18.8,2.5));
#7357=CARTESIAN_POINT('',(-8.,18.8,2.5));
#7358=CARTESIAN_POINT('Origin',(-9.,18.8,2.5));
#7359=CARTESIAN_POINT('',(8.00000000000001,18.8,2.5));
#7360=CARTESIAN_POINT('Origin',(0.,18.8,2.5));
#7361=CARTESIAN_POINT('Origin',(9.00000000000001,18.8,2.5));
#7362=CARTESIAN_POINT('Origin',(-1.73472347597681E-15,18.8,-2.5));
#7363=CARTESIAN_POINT('',(8.,18.8,-2.5));
#7364=CARTESIAN_POINT('Origin',(9.,18.8,-2.5));
#7365=CARTESIAN_POINT('',(-8.,18.8,-2.5));
#7366=CARTESIAN_POINT('Origin',(-1.73472347597681E-15,18.8,-2.5));
#7367=CARTESIAN_POINT('Origin',(-9.,18.8,-2.5));
#7368=CARTESIAN_POINT('Origin',(-9.,18.8,2.5));
#7369=CARTESIAN_POINT('',(-8.,18.8,2.5));
#7370=CARTESIAN_POINT('Origin',(9.,18.8,-2.5));
#7371=CARTESIAN_POINT('',(8.,18.8,-2.5));
#7372=CARTESIAN_POINT('Origin',(0.,16.6,2.5));
#7373=CARTESIAN_POINT('',(-8.,16.6,2.5));
#7374=CARTESIAN_POINT('Origin',(-9.,16.6,2.5));
#7375=CARTESIAN_POINT('',(8.00000000000001,16.6,2.5));
#7376=CARTESIAN_POINT('Origin',(0.,16.6,2.5));
#7377=CARTESIAN_POINT('Origin',(9.00000000000001,16.6,2.5));
#7378=CARTESIAN_POINT('Origin',(-1.73472347597681E-15,16.6,-2.5));
#7379=CARTESIAN_POINT('',(8.,16.6,-2.5));
#7380=CARTESIAN_POINT('Origin',(9.,16.6,-2.5));
#7381=CARTESIAN_POINT('',(-8.,16.6,-2.5));
#7382=CARTESIAN_POINT('Origin',(-1.73472347597681E-15,16.6,-2.5));
#7383=CARTESIAN_POINT('Origin',(-9.,16.6,-2.5));
#7384=CARTESIAN_POINT('Origin',(-9.,16.6,2.5));
#7385=CARTESIAN_POINT('',(-8.,16.6,2.5));
#7386=CARTESIAN_POINT('Origin',(9.,16.6,-2.5));
#7387=CARTESIAN_POINT('',(8.,16.6,-2.5));
#7613=UNCERTAINTY_MEASURE_WITH_UNIT(LENGTH_MEASURE(0.01),#7628,
'DISTANCE_ACCURACY_VALUE',
'Maximum model space distance between geometric entities at asserted c
onnectivities');
#7616=UNCERTAINTY_MEASURE_WITH_UNIT(LENGTH_MEASURE(0.01),#7628,
'DISTANCE_ACCURACY_VALUE',
'Maximum model space distance between geometric entities at asserted c
onnectivities');
#7624=(
GEOMETRIC_REPRESENTATION_CONTEXT(3)
GLOBAL_UNCERTAINTY_ASSIGNED_CONTEXT((#7613))
GLOBAL_UNIT_ASSIGNED_CONTEXT((#7628,#7630,#7631))
REPRESENTATION_CONTEXT('','3D')
);
#7627=(
GEOMETRIC_REPRESENTATION_CONTEXT(3)
GLOBAL_UNCERTAINTY_ASSIGNED_CONTEXT((#7616))
GLOBAL_UNIT_ASSIGNED_CONTEXT((#7628,#7630,#7631))
REPRESENTATION_CONTEXT('','3D')
);
#7628=(
LENGTH_UNIT()
NAMED_UNIT(*)
SI_UNIT(.MILLI.,.METRE.)
);
#7630=(
NAMED_UNIT(*)
PLANE_ANGLE_UNIT()
SI_UNIT($,.RADIAN.)
);
#7631=(
NAMED_UNIT(*)
SI_UNIT($,.STERADIAN.)
SOLID_ANGLE_UNIT()
);
#7639=SHAPE_DEFINITION_REPRESENTATION(#7649,#7671);
#7649=PRODUCT_DEFINITION_SHAPE('',$,#7682);
#7671=SHAPE_REPRESENTATION('',(#2645),#7624);
#7674=PRODUCT_DEFINITION_CONTEXT('part definition',#7706,'design');
#7682=PRODUCT_DEFINITION('coil','coil',#7692,#7674);
#7692=PRODUCT_DEFINITION_FORMATION('',$,#7715);
#7706=APPLICATION_CONTEXT(
'Core Data for Automotive Mechanical Design Process');
#7707=PRODUCT_CONTEXT('part definition',#7706,'mechanical');
#7715=PRODUCT('coil','coil',$,(#7707));
#7723=PRESENTATION_STYLE_ASSIGNMENT((#7729));
#7729=SURFACE_STYLE_USAGE(.BOTH.,#7735);
#7735=SURFACE_SIDE_STYLE('',(#7741));
#7741=SURFACE_STYLE_FILL_AREA(#7747);
#7747=FILL_AREA_STYLE('Opaque(97,158,199)',(#7753));
#7753=FILL_AREA_STYLE_COLOUR('Opaque(97,158,199)',#7759);
#7759=COLOUR_RGB('Opaque(97,158,199)',0.380392156862745,0.619607843137255,
0.780392156862745);
ENDSEC;
END-ISO-10303-21;
